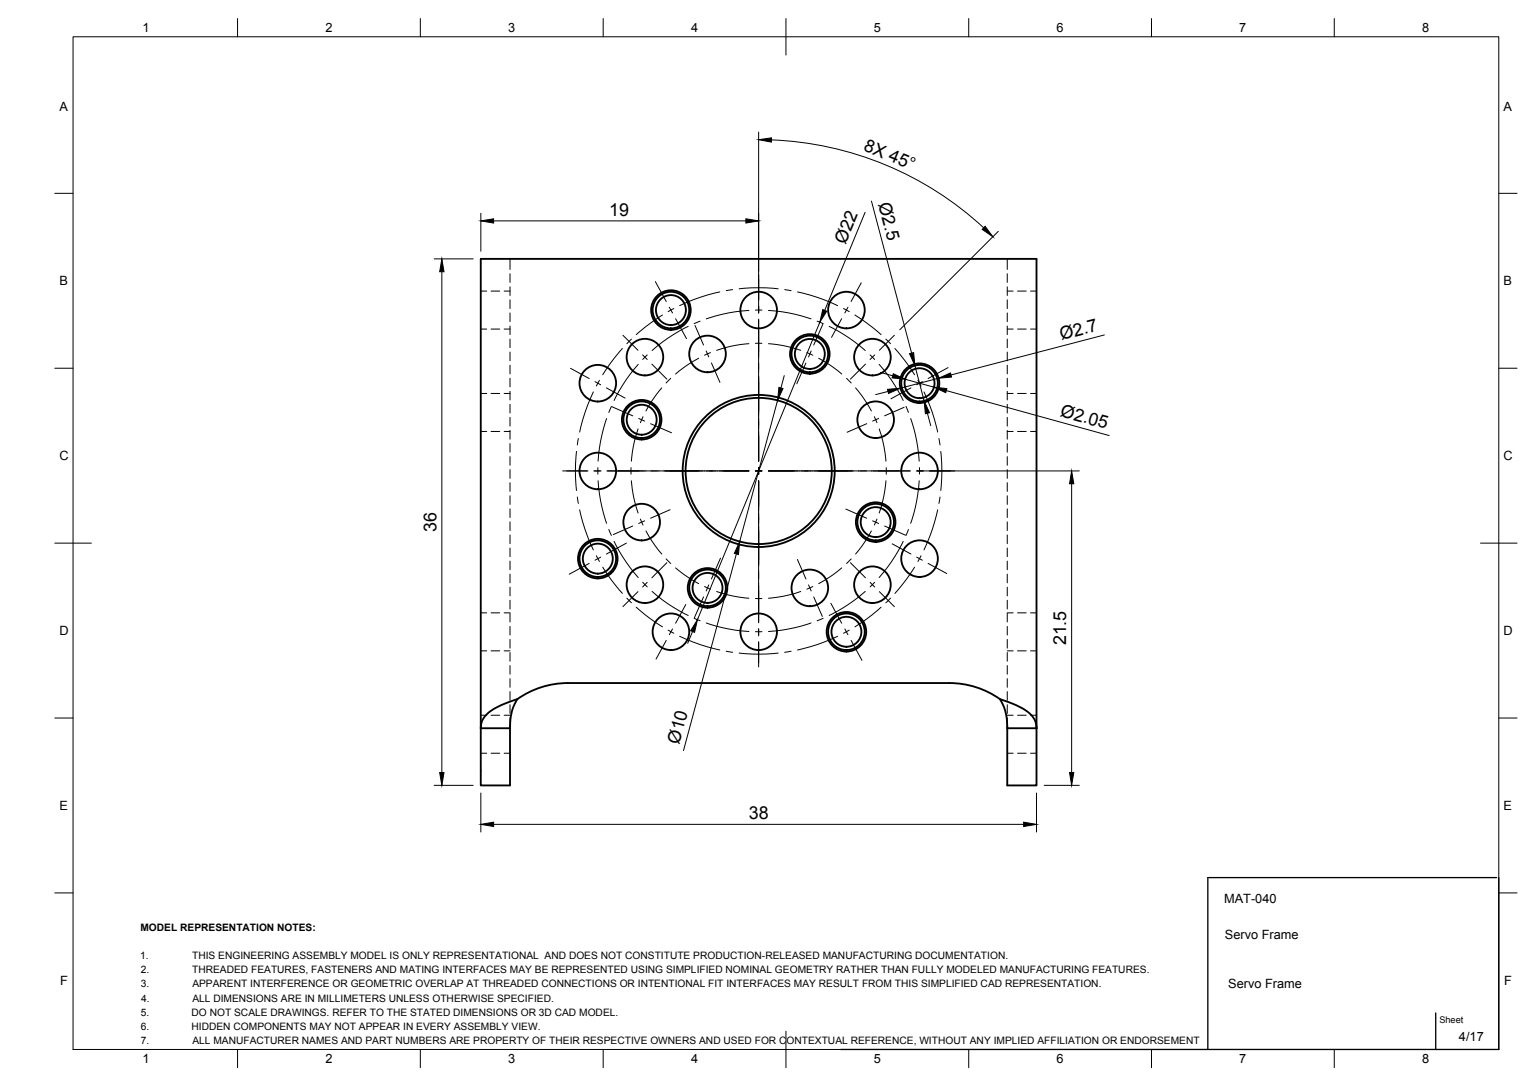
ISO-10303-21;
HEADER;
/* Generated by software containing ST-Developer
 * from STEP Tools, Inc. (www.steptools.com) 
 */

FILE_DESCRIPTION(
/* description */ ('STEP AP214'),
/* implementation_level */ '2;1');

FILE_NAME(
/* name */ 'Servo Frame.step',
/* time_stamp */ '2026-11-14T21:53:28-08:00',
/* author */ (''),
/* organization */ (''),
/* preprocessor_version */ 'ST-DEVELOPER v20.2',
/* originating_system */ 'Autodesk Translation Framework v15.17.0.0',
/* authorisation */ '');

FILE_SCHEMA (('AUTOMOTIVE_DESIGN { 1 0 10303 214 3 1 1 }'));
ENDSEC;

DATA;
#10=MECHANICAL_DESIGN_GEOMETRIC_PRESENTATION_REPRESENTATION('',(#320,#321,#322,#323,#324,#325,#326,#327,#328),#20176);
#187=OPEN_SHELL('',(#10781));
#188=OPEN_SHELL('',(#10782));
#189=OPEN_SHELL('',(#10783));
#190=OPEN_SHELL('',(#10784));
#191=OPEN_SHELL('',(#10785));
#192=OPEN_SHELL('',(#10786));
#193=OPEN_SHELL('',(#10787));
#194=OPEN_SHELL('',(#10788));
#195=SHELL_BASED_SURFACE_MODEL('Body2',(#187));
#196=SHELL_BASED_SURFACE_MODEL('Body3',(#188));
#197=SHELL_BASED_SURFACE_MODEL('Body4',(#189));
#198=SHELL_BASED_SURFACE_MODEL('Body5',(#190));
#199=SHELL_BASED_SURFACE_MODEL('Body6',(#191));
#200=SHELL_BASED_SURFACE_MODEL('Body7',(#192));
#201=SHELL_BASED_SURFACE_MODEL('Body8',(#193));
#202=SHELL_BASED_SURFACE_MODEL('Body9',(#194));
#203=ELLIPSE('',#11797,7.14648376237048,6.18893462761436);
#204=ELLIPSE('',#11803,7.14646345436459,6.18889945302544);
#205=CONICAL_SURFACE('',#11750,1.34999999991669,0.785398163397448);
#206=CONICAL_SURFACE('',#11752,1.34999999991669,0.785398163397448);
#207=CONICAL_SURFACE('',#11754,1.34999999991669,0.785398163397448);
#208=CONICAL_SURFACE('',#11756,1.34999999991669,0.785398163397448);
#209=CONICAL_SURFACE('',#11758,1.34999999990714,0.785398163397448);
#210=CONICAL_SURFACE('',#11760,1.34999999990714,0.785398163397448);
#211=CONICAL_SURFACE('',#11762,1.34999999990714,0.785398163397448);
#212=CONICAL_SURFACE('',#11764,1.34999999990714,0.785398163397448);
#213=CONICAL_SURFACE('',#11766,5.19997115839037,0.785393345879516);
#240=B_SPLINE_SURFACE_WITH_KNOTS('',3,3,((#19092,#19093,#19094,#19095),
(#19096,#19097,#19098,#19099),(#19100,#19101,#19102,#19103),(#19104,#19105,
#19106,#19107),(#19108,#19109,#19110,#19111),(#19112,#19113,#19114,#19115),
(#19116,#19117,#19118,#19119),(#19120,#19121,#19122,#19123),(#19124,#19125,
#19126,#19127)),.UNSPECIFIED.,.F.,.F.,.F.,(4,1,1,1,1,1,4),(4,4),(-0.01838458257717,
0.,0.25,0.5,0.75,1.,1.018710256812),(-0.03706965294501,1.037304298792),
 .UNSPECIFIED.);
#241=B_SPLINE_SURFACE_WITH_KNOTS('',3,3,((#19144,#19145,#19146,#19147),
(#19148,#19149,#19150,#19151),(#19152,#19153,#19154,#19155),(#19156,#19157,
#19158,#19159),(#19160,#19161,#19162,#19163),(#19164,#19165,#19166,#19167),
(#19168,#19169,#19170,#19171),(#19172,#19173,#19174,#19175),(#19176,#19177,
#19178,#19179)),.UNSPECIFIED.,.F.,.F.,.F.,(4,1,1,1,1,1,4),(4,4),(-0.01864501026175,
0.,0.25,0.5,0.75,1.,1.018470834436),(-0.03706965294501,1.037304298792),
 .UNSPECIFIED.);
#242=B_SPLINE_SURFACE_WITH_KNOTS('',3,3,((#19239,#19240,#19241,#19242),
(#19243,#19244,#19245,#19246),(#19247,#19248,#19249,#19250),(#19251,#19252,
#19253,#19254),(#19255,#19256,#19257,#19258),(#19259,#19260,#19261,#19262)),
 .UNSPECIFIED.,.F.,.F.,.F.,(4,1,1,4),(4,4),(-0.7776806408489,0.,1.,1.777680640849),
(-0.03706965294501,1.037069667454),.UNSPECIFIED.);
#243=B_SPLINE_SURFACE_WITH_KNOTS('',3,3,((#19263,#19264,#19265,#19266),
(#19267,#19268,#19269,#19270),(#19271,#19272,#19273,#19274),(#19275,#19276,
#19277,#19278),(#19279,#19280,#19281,#19282),(#19283,#19284,#19285,#19286)),
 .UNSPECIFIED.,.F.,.F.,.F.,(4,1,1,4),(4,4),(-0.7776806408488,0.,1.,1.777680640849),
(-0.03706965294501,1.037069667454),.UNSPECIFIED.);
#288=B_SPLINE_CURVE_WITH_KNOTS('',3,(#19003,#19004,#19005,#19006,#19007,
#19008,#19009,#19010,#19011,#19012,#19013,#19014,#19015,#19016),
 .UNSPECIFIED.,.F.,.F.,(4,2,2,2,2,2,4),(1.0000000090833E-6,0.0397704331538061,
0.0783295476556165,0.10311510516028,0.130769699028325,0.170261252779255,
0.207364811990595),.UNSPECIFIED.);
#289=B_SPLINE_CURVE_WITH_KNOTS('',3,(#19045,#19046,#19047,#19048,#19049,
#19050,#19051,#19052,#19053,#19054,#19055,#19056,#19057,#19058),
 .UNSPECIFIED.,.F.,.F.,(4,2,2,2,2,2,4),(1.00000005137352E-6,0.0364150080452644,
0.0751701681205766,0.102306577132939,0.126714048144896,0.164687443503408,
0.20385265381537),.UNSPECIFIED.);
#290=B_SPLINE_CURVE_WITH_KNOTS('',3,(#19129,#19130,#19131,#19132,#19133,
#19134,#19135,#19136,#19137,#19138,#19139,#19140,#19141,#19142),
 .UNSPECIFIED.,.F.,.F.,(4,2,2,2,2,2,4),(1.00000002985316E-6,0.0497274416726429,
0.101777541549185,0.213706159601663,0.317575823833734,0.371841554247195,
0.427578702498277),.UNSPECIFIED.);
#291=B_SPLINE_CURVE_WITH_KNOTS('',3,(#19182,#19183,#19184,#19185,#19186,
#19187,#19188,#19189,#19190,#19191,#19192,#19193,#19194,#19195),
 .UNSPECIFIED.,.F.,.F.,(4,2,2,2,2,2,4),(1.00000005253209E-6,0.0558510119021626,
0.110229405327848,0.214323647321834,0.326650579970185,0.379079827251892,
0.429160855957136),.UNSPECIFIED.);
#296=SHAPE_REPRESENTATION_RELATIONSHIP('SRR','None',#20258,#308);
#308=ADVANCED_BREP_SHAPE_REPRESENTATION('',(#355),#20164);
#320=STYLED_ITEM('',(#20334),#355);
#321=STYLED_ITEM('',(#20334),#195);
#322=STYLED_ITEM('',(#20334),#196);
#323=STYLED_ITEM('',(#20334),#197);
#324=STYLED_ITEM('',(#20334),#198);
#325=STYLED_ITEM('',(#20334),#199);
#326=STYLED_ITEM('',(#20334),#200);
#327=STYLED_ITEM('',(#20334),#201);
#328=STYLED_ITEM('',(#20334),#202);
#355=MANIFOLD_SOLID_BREP('Body1',#10946);
#450=FACE_BOUND('',#1962,.T.);
#451=FACE_BOUND('',#1963,.T.);
#452=FACE_BOUND('',#1964,.T.);
#453=FACE_BOUND('',#1965,.T.);
#454=FACE_BOUND('',#1966,.T.);
#455=FACE_BOUND('',#1967,.T.);
#456=FACE_BOUND('',#1968,.T.);
#457=FACE_BOUND('',#1969,.T.);
#458=FACE_BOUND('',#1970,.T.);
#459=FACE_BOUND('',#1971,.T.);
#460=FACE_BOUND('',#1972,.T.);
#461=FACE_BOUND('',#1973,.T.);
#462=FACE_BOUND('',#1974,.T.);
#463=FACE_BOUND('',#1975,.T.);
#464=FACE_BOUND('',#1976,.T.);
#465=FACE_BOUND('',#1977,.T.);
#466=FACE_BOUND('',#1978,.T.);
#467=FACE_BOUND('',#1979,.T.);
#468=FACE_BOUND('',#1980,.T.);
#469=FACE_BOUND('',#1981,.T.);
#470=FACE_BOUND('',#1982,.T.);
#471=FACE_BOUND('',#1983,.T.);
#472=FACE_BOUND('',#1984,.T.);
#473=FACE_BOUND('',#1985,.T.);
#474=FACE_BOUND('',#1986,.T.);
#475=FACE_BOUND('',#1994,.T.);
#476=FACE_BOUND('',#1995,.T.);
#477=FACE_BOUND('',#1996,.T.);
#478=FACE_BOUND('',#1997,.T.);
#479=FACE_BOUND('',#1998,.T.);
#480=FACE_BOUND('',#1999,.T.);
#481=FACE_BOUND('',#2000,.T.);
#482=FACE_BOUND('',#2001,.T.);
#483=FACE_BOUND('',#2002,.T.);
#484=FACE_BOUND('',#2003,.T.);
#485=FACE_BOUND('',#2004,.T.);
#486=FACE_BOUND('',#2005,.T.);
#487=FACE_BOUND('',#2006,.T.);
#488=FACE_BOUND('',#2007,.T.);
#489=FACE_BOUND('',#2008,.T.);
#490=FACE_BOUND('',#2009,.T.);
#491=FACE_BOUND('',#2010,.T.);
#492=FACE_BOUND('',#2011,.T.);
#493=FACE_BOUND('',#2012,.T.);
#494=FACE_BOUND('',#2013,.T.);
#495=FACE_BOUND('',#2014,.T.);
#496=FACE_BOUND('',#2015,.T.);
#497=FACE_BOUND('',#2016,.T.);
#498=FACE_BOUND('',#2017,.T.);
#499=FACE_BOUND('',#2018,.T.);
#500=FACE_BOUND('',#2020,.T.);
#501=FACE_BOUND('',#2021,.T.);
#502=FACE_BOUND('',#2022,.T.);
#503=FACE_BOUND('',#2023,.T.);
#504=FACE_BOUND('',#2027,.T.);
#505=FACE_BOUND('',#2028,.T.);
#506=FACE_BOUND('',#2029,.T.);
#507=FACE_BOUND('',#2030,.T.);
#508=FACE_BOUND('',#2046,.T.);
#509=FACE_BOUND('',#2047,.T.);
#510=FACE_BOUND('',#2048,.T.);
#511=FACE_BOUND('',#2049,.T.);
#512=FACE_BOUND('',#2051,.T.);
#513=FACE_BOUND('',#2052,.T.);
#514=FACE_BOUND('',#2053,.T.);
#515=FACE_BOUND('',#2054,.T.);
#808=PLANE('',#11792);
#809=PLANE('',#11798);
#810=PLANE('',#11806);
#811=PLANE('',#11809);
#812=PLANE('',#11810);
#813=PLANE('',#11814);
#814=PLANE('',#11822);
#815=PLANE('',#11827);
#816=PLANE('',#11830);
#817=PLANE('',#11835);
#818=PLANE('',#11838);
#819=PLANE('',#11839);
#820=PLANE('',#11840);
#821=PLANE('',#11841);
#1257=FACE_OUTER_BOUND('',#1919,.T.);
#1258=FACE_OUTER_BOUND('',#1920,.T.);
#1259=FACE_OUTER_BOUND('',#1921,.T.);
#1260=FACE_OUTER_BOUND('',#1922,.T.);
#1261=FACE_OUTER_BOUND('',#1923,.T.);
#1262=FACE_OUTER_BOUND('',#1924,.T.);
#1263=FACE_OUTER_BOUND('',#1925,.T.);
#1264=FACE_OUTER_BOUND('',#1926,.T.);
#1265=FACE_OUTER_BOUND('',#1927,.T.);
#1266=FACE_OUTER_BOUND('',#1928,.T.);
#1267=FACE_OUTER_BOUND('',#1929,.T.);
#1268=FACE_OUTER_BOUND('',#1930,.T.);
#1269=FACE_OUTER_BOUND('',#1931,.T.);
#1270=FACE_OUTER_BOUND('',#1932,.T.);
#1271=FACE_OUTER_BOUND('',#1933,.T.);
#1272=FACE_OUTER_BOUND('',#1934,.T.);
#1273=FACE_OUTER_BOUND('',#1935,.T.);
#1274=FACE_OUTER_BOUND('',#1936,.T.);
#1275=FACE_OUTER_BOUND('',#1937,.T.);
#1276=FACE_OUTER_BOUND('',#1938,.T.);
#1277=FACE_OUTER_BOUND('',#1939,.T.);
#1278=FACE_OUTER_BOUND('',#1940,.T.);
#1279=FACE_OUTER_BOUND('',#1941,.T.);
#1280=FACE_OUTER_BOUND('',#1942,.T.);
#1281=FACE_OUTER_BOUND('',#1943,.T.);
#1282=FACE_OUTER_BOUND('',#1944,.T.);
#1283=FACE_OUTER_BOUND('',#1945,.T.);
#1284=FACE_OUTER_BOUND('',#1946,.T.);
#1285=FACE_OUTER_BOUND('',#1947,.T.);
#1286=FACE_OUTER_BOUND('',#1948,.T.);
#1287=FACE_OUTER_BOUND('',#1949,.T.);
#1288=FACE_OUTER_BOUND('',#1950,.T.);
#1289=FACE_OUTER_BOUND('',#1951,.T.);
#1290=FACE_OUTER_BOUND('',#1952,.T.);
#1291=FACE_OUTER_BOUND('',#1953,.T.);
#1292=FACE_OUTER_BOUND('',#1954,.T.);
#1293=FACE_OUTER_BOUND('',#1955,.T.);
#1294=FACE_OUTER_BOUND('',#1956,.T.);
#1295=FACE_OUTER_BOUND('',#1957,.T.);
#1296=FACE_OUTER_BOUND('',#1958,.T.);
#1297=FACE_OUTER_BOUND('',#1959,.T.);
#1298=FACE_OUTER_BOUND('',#1960,.T.);
#1299=FACE_OUTER_BOUND('',#1961,.T.);
#1300=FACE_OUTER_BOUND('',#1987,.T.);
#1301=FACE_OUTER_BOUND('',#1988,.T.);
#1302=FACE_OUTER_BOUND('',#1989,.T.);
#1303=FACE_OUTER_BOUND('',#1990,.T.);
#1304=FACE_OUTER_BOUND('',#1991,.T.);
#1305=FACE_OUTER_BOUND('',#1992,.T.);
#1306=FACE_OUTER_BOUND('',#1993,.T.);
#1307=FACE_OUTER_BOUND('',#2019,.T.);
#1308=FACE_OUTER_BOUND('',#2024,.T.);
#1309=FACE_OUTER_BOUND('',#2025,.T.);
#1310=FACE_OUTER_BOUND('',#2026,.T.);
#1311=FACE_OUTER_BOUND('',#2031,.T.);
#1312=FACE_OUTER_BOUND('',#2032,.T.);
#1313=FACE_OUTER_BOUND('',#2033,.T.);
#1314=FACE_OUTER_BOUND('',#2034,.T.);
#1315=FACE_OUTER_BOUND('',#2035,.T.);
#1316=FACE_OUTER_BOUND('',#2036,.T.);
#1317=FACE_OUTER_BOUND('',#2037,.T.);
#1318=FACE_OUTER_BOUND('',#2038,.T.);
#1319=FACE_OUTER_BOUND('',#2039,.T.);
#1320=FACE_OUTER_BOUND('',#2040,.T.);
#1321=FACE_OUTER_BOUND('',#2041,.T.);
#1322=FACE_OUTER_BOUND('',#2042,.T.);
#1323=FACE_OUTER_BOUND('',#2043,.T.);
#1324=FACE_OUTER_BOUND('',#2044,.T.);
#1325=FACE_OUTER_BOUND('',#2045,.T.);
#1326=FACE_OUTER_BOUND('',#2050,.T.);
#1327=FACE_OUTER_BOUND('',#2055,.T.);
#1328=FACE_OUTER_BOUND('',#2056,.T.);
#1329=FACE_OUTER_BOUND('',#2057,.T.);
#1330=FACE_OUTER_BOUND('',#2058,.T.);
#1331=FACE_OUTER_BOUND('',#2059,.T.);
#1332=FACE_OUTER_BOUND('',#2060,.T.);
#1333=FACE_OUTER_BOUND('',#2061,.T.);
#1334=FACE_OUTER_BOUND('',#2062,.T.);
#1335=FACE_OUTER_BOUND('',#2063,.T.);
#1336=FACE_OUTER_BOUND('',#2064,.T.);
#1919=EDGE_LOOP('',(#9045,#9046,#9047,#9048));
#1920=EDGE_LOOP('',(#9049,#9050,#9051,#9052));
#1921=EDGE_LOOP('',(#9053,#9054,#9055,#9056));
#1922=EDGE_LOOP('',(#9057,#9058,#9059,#9060));
#1923=EDGE_LOOP('',(#9061,#9062,#9063,#9064));
#1924=EDGE_LOOP('',(#9065,#9066,#9067,#9068));
#1925=EDGE_LOOP('',(#9069,#9070,#9071,#9072));
#1926=EDGE_LOOP('',(#9073,#9074,#9075,#9076));
#1927=EDGE_LOOP('',(#9077,#9078,#9079,#9080));
#1928=EDGE_LOOP('',(#9081,#9082,#9083,#9084));
#1929=EDGE_LOOP('',(#9085,#9086,#9087,#9088));
#1930=EDGE_LOOP('',(#9089,#9090,#9091,#9092));
#1931=EDGE_LOOP('',(#9093,#9094,#9095,#9096));
#1932=EDGE_LOOP('',(#9097,#9098,#9099,#9100));
#1933=EDGE_LOOP('',(#9101,#9102,#9103,#9104));
#1934=EDGE_LOOP('',(#9105,#9106,#9107,#9108));
#1935=EDGE_LOOP('',(#9109,#9110,#9111,#9112));
#1936=EDGE_LOOP('',(#9113,#9114,#9115,#9116));
#1937=EDGE_LOOP('',(#9117,#9118,#9119,#9120));
#1938=EDGE_LOOP('',(#9121,#9122,#9123,#9124));
#1939=EDGE_LOOP('',(#9125,#9126,#9127,#9128));
#1940=EDGE_LOOP('',(#9129,#9130,#9131,#9132));
#1941=EDGE_LOOP('',(#9133,#9134,#9135,#9136));
#1942=EDGE_LOOP('',(#9137,#9138,#9139,#9140));
#1943=EDGE_LOOP('',(#9141,#9142,#9143,#9144));
#1944=EDGE_LOOP('',(#9145,#9146,#9147,#9148));
#1945=EDGE_LOOP('',(#9149,#9150,#9151,#9152));
#1946=EDGE_LOOP('',(#9153,#9154,#9155,#9156));
#1947=EDGE_LOOP('',(#9157,#9158,#9159,#9160));
#1948=EDGE_LOOP('',(#9161,#9162,#9163,#9164));
#1949=EDGE_LOOP('',(#9165,#9166,#9167,#9168));
#1950=EDGE_LOOP('',(#9169,#9170,#9171,#9172));
#1951=EDGE_LOOP('',(#9173,#9174,#9175,#9176));
#1952=EDGE_LOOP('',(#9177,#9178,#9179,#9180));
#1953=EDGE_LOOP('',(#9181,#9182,#9183,#9184));
#1954=EDGE_LOOP('',(#9185,#9186,#9187,#9188));
#1955=EDGE_LOOP('',(#9189,#9190,#9191,#9192));
#1956=EDGE_LOOP('',(#9193,#9194,#9195,#9196));
#1957=EDGE_LOOP('',(#9197,#9198,#9199,#9200));
#1958=EDGE_LOOP('',(#9201,#9202,#9203,#9204));
#1959=EDGE_LOOP('',(#9205,#9206,#9207,#9208));
#1960=EDGE_LOOP('',(#9209,#9210,#9211,#9212));
#1961=EDGE_LOOP('',(#9213,#9214,#9215,#9216,#9217,#9218));
#1962=EDGE_LOOP('',(#9219));
#1963=EDGE_LOOP('',(#9220));
#1964=EDGE_LOOP('',(#9221));
#1965=EDGE_LOOP('',(#9222));
#1966=EDGE_LOOP('',(#9223));
#1967=EDGE_LOOP('',(#9224));
#1968=EDGE_LOOP('',(#9225));
#1969=EDGE_LOOP('',(#9226));
#1970=EDGE_LOOP('',(#9227));
#1971=EDGE_LOOP('',(#9228));
#1972=EDGE_LOOP('',(#9229));
#1973=EDGE_LOOP('',(#9230));
#1974=EDGE_LOOP('',(#9231));
#1975=EDGE_LOOP('',(#9232));
#1976=EDGE_LOOP('',(#9233));
#1977=EDGE_LOOP('',(#9234));
#1978=EDGE_LOOP('',(#9235));
#1979=EDGE_LOOP('',(#9236));
#1980=EDGE_LOOP('',(#9237));
#1981=EDGE_LOOP('',(#9238));
#1982=EDGE_LOOP('',(#9239));
#1983=EDGE_LOOP('',(#9240));
#1984=EDGE_LOOP('',(#9241));
#1985=EDGE_LOOP('',(#9242));
#1986=EDGE_LOOP('',(#9243));
#1987=EDGE_LOOP('',(#9244,#9245,#9246,#9247,#9248));
#1988=EDGE_LOOP('',(#9249,#9250,#9251,#9252,#9253,#9254,#9255,#9256,#9257,
#9258,#9259,#9260));
#1989=EDGE_LOOP('',(#9261,#9262,#9263,#9264,#9265));
#1990=EDGE_LOOP('',(#9266,#9267,#9268,#9269,#9270));
#1991=EDGE_LOOP('',(#9271,#9272,#9273,#9274));
#1992=EDGE_LOOP('',(#9275,#9276,#9277,#9278,#9279));
#1993=EDGE_LOOP('',(#9280,#9281,#9282,#9283,#9284,#9285));
#1994=EDGE_LOOP('',(#9286));
#1995=EDGE_LOOP('',(#9287));
#1996=EDGE_LOOP('',(#9288));
#1997=EDGE_LOOP('',(#9289));
#1998=EDGE_LOOP('',(#9290));
#1999=EDGE_LOOP('',(#9291));
#2000=EDGE_LOOP('',(#9292));
#2001=EDGE_LOOP('',(#9293));
#2002=EDGE_LOOP('',(#9294));
#2003=EDGE_LOOP('',(#9295));
#2004=EDGE_LOOP('',(#9296));
#2005=EDGE_LOOP('',(#9297));
#2006=EDGE_LOOP('',(#9298));
#2007=EDGE_LOOP('',(#9299));
#2008=EDGE_LOOP('',(#9300));
#2009=EDGE_LOOP('',(#9301));
#2010=EDGE_LOOP('',(#9302));
#2011=EDGE_LOOP('',(#9303));
#2012=EDGE_LOOP('',(#9304));
#2013=EDGE_LOOP('',(#9305));
#2014=EDGE_LOOP('',(#9306));
#2015=EDGE_LOOP('',(#9307));
#2016=EDGE_LOOP('',(#9308));
#2017=EDGE_LOOP('',(#9309));
#2018=EDGE_LOOP('',(#9310));
#2019=EDGE_LOOP('',(#9311,#9312,#9313,#9314,#9315,#9316,#9317,#9318));
#2020=EDGE_LOOP('',(#9319));
#2021=EDGE_LOOP('',(#9320));
#2022=EDGE_LOOP('',(#9321));
#2023=EDGE_LOOP('',(#9322));
#2024=EDGE_LOOP('',(#9323,#9324,#9325,#9326,#9327));
#2025=EDGE_LOOP('',(#9328,#9329,#9330,#9331,#9332));
#2026=EDGE_LOOP('',(#9333,#9334,#9335,#9336,#9337,#9338,#9339,#9340));
#2027=EDGE_LOOP('',(#9341));
#2028=EDGE_LOOP('',(#9342));
#2029=EDGE_LOOP('',(#9343));
#2030=EDGE_LOOP('',(#9344));
#2031=EDGE_LOOP('',(#9345,#9346,#9347,#9348,#9349));
#2032=EDGE_LOOP('',(#9350,#9351,#9352,#9353,#9354));
#2033=EDGE_LOOP('',(#9355,#9356,#9357,#9358,#9359));
#2034=EDGE_LOOP('',(#9360,#9361,#9362,#9363));
#2035=EDGE_LOOP('',(#9364,#9365,#9366,#9367));
#2036=EDGE_LOOP('',(#9368,#9369,#9370,#9371));
#2037=EDGE_LOOP('',(#9372,#9373,#9374,#9375));
#2038=EDGE_LOOP('',(#9376,#9377,#9378,#9379,#9380));
#2039=EDGE_LOOP('',(#9381,#9382,#9383,#9384,#9385));
#2040=EDGE_LOOP('',(#9386,#9387,#9388,#9389));
#2041=EDGE_LOOP('',(#9390,#9391,#9392,#9393));
#2042=EDGE_LOOP('',(#9394,#9395,#9396,#9397));
#2043=EDGE_LOOP('',(#9398,#9399,#9400,#9401,#9402));
#2044=EDGE_LOOP('',(#9403,#9404,#9405,#9406));
#2045=EDGE_LOOP('',(#9407,#9408,#9409,#9410,#9411,#9412,#9413,#9414));
#2046=EDGE_LOOP('',(#9415));
#2047=EDGE_LOOP('',(#9416));
#2048=EDGE_LOOP('',(#9417));
#2049=EDGE_LOOP('',(#9418));
#2050=EDGE_LOOP('',(#9419,#9420,#9421,#9422,#9423,#9424,#9425,#9426));
#2051=EDGE_LOOP('',(#9427));
#2052=EDGE_LOOP('',(#9428));
#2053=EDGE_LOOP('',(#9429));
#2054=EDGE_LOOP('',(#9430));
#2055=EDGE_LOOP('',(#9431,#9432,#9433,#9434));
#2056=EDGE_LOOP('',(#9435,#9436,#9437,#9438));
#2057=EDGE_LOOP('',(#9439,#9440,#9441,#9442));
#2058=EDGE_LOOP('',(#9443,#9444,#9445,#9446));
#2059=EDGE_LOOP('',(#9447,#9448,#9449,#9450));
#2060=EDGE_LOOP('',(#9451,#9452,#9453,#9454));
#2061=EDGE_LOOP('',(#9455,#9456,#9457,#9458));
#2062=EDGE_LOOP('',(#9459,#9460,#9461,#9462));
#2063=EDGE_LOOP('',(#9463,#9464,#9465,#9466));
#2064=EDGE_LOOP('',(#9467,#9468,#9469,#9470));
#2967=LINE('',#18756,#3955);
#2968=LINE('',#18762,#3956);
#2969=LINE('',#18768,#3957);
#2970=LINE('',#18774,#3958);
#2971=LINE('',#18780,#3959);
#2972=LINE('',#18786,#3960);
#2973=LINE('',#18792,#3961);
#2974=LINE('',#18798,#3962);
#2975=LINE('',#18804,#3963);
#2976=LINE('',#18810,#3964);
#2977=LINE('',#18816,#3965);
#2978=LINE('',#18822,#3966);
#2979=LINE('',#18828,#3967);
#2980=LINE('',#18834,#3968);
#2981=LINE('',#18840,#3969);
#2982=LINE('',#18846,#3970);
#2983=LINE('',#18852,#3971);
#2984=LINE('',#18858,#3972);
#2985=LINE('',#18864,#3973);
#2986=LINE('',#18870,#3974);
#2987=LINE('',#18876,#3975);
#2988=LINE('',#18882,#3976);
#2989=LINE('',#18888,#3977);
#2990=LINE('',#18894,#3978);
#2991=LINE('',#18900,#3979);
#2992=LINE('',#18904,#3980);
#2993=LINE('',#18908,#3981);
#2994=LINE('',#18912,#3982);
#2995=LINE('',#18916,#3983);
#2996=LINE('',#18920,#3984);
#2997=LINE('',#18924,#3985);
#2998=LINE('',#18928,#3986);
#2999=LINE('',#18932,#3987);
#3000=LINE('',#18936,#3988);
#3001=LINE('',#18942,#3989);
#3002=LINE('',#18948,#3990);
#3003=LINE('',#18954,#3991);
#3004=LINE('',#18960,#3992);
#3005=LINE('',#18966,#3993);
#3006=LINE('',#18972,#3994);
#3007=LINE('',#18978,#3995);
#3008=LINE('',#18984,#3996);
#3009=LINE('',#18989,#3997);
#3010=LINE('',#18991,#3998);
#3011=LINE('',#18995,#3999);
#3012=LINE('',#18998,#4000);
#3013=LINE('',#19019,#4001);
#3014=LINE('',#19022,#4002);
#3015=LINE('',#19024,#4003);
#3016=LINE('',#19026,#4004);
#3017=LINE('',#19030,#4005);
#3018=LINE('',#19034,#4006);
#3019=LINE('',#19036,#4007);
#3020=LINE('',#19038,#4008);
#3021=LINE('',#19042,#4009);
#3022=LINE('',#19061,#4010);
#3023=LINE('',#19063,#4011);
#3024=LINE('',#19066,#4012);
#3025=LINE('',#19069,#4013);
#3026=LINE('',#19070,#4014);
#3027=LINE('',#19075,#4015);
#3028=LINE('',#19076,#4016);
#3029=LINE('',#19078,#4017);
#3030=LINE('',#19079,#4018);
#3031=LINE('',#19082,#4019);
#3032=LINE('',#19086,#4020);
#3033=LINE('',#19090,#4021);
#3034=LINE('',#19143,#4022);
#3035=LINE('',#19181,#4023);
#3036=LINE('',#19201,#4024);
#3037=LINE('',#19204,#4025);
#3038=LINE('',#19207,#4026);
#3039=LINE('',#19210,#4027);
#3040=LINE('',#19215,#4028);
#3041=LINE('',#19218,#4029);
#3042=LINE('',#19219,#4030);
#3043=LINE('',#19221,#4031);
#3044=LINE('',#19222,#4032);
#3045=LINE('',#19226,#4033);
#3046=LINE('',#19229,#4034);
#3047=LINE('',#19232,#4035);
#3048=LINE('',#19235,#4036);
#3049=LINE('',#19236,#4037);
#3050=LINE('',#19288,#4038);
#3051=LINE('',#19289,#4039);
#3052=LINE('',#19292,#4040);
#3053=LINE('',#19294,#4041);
#3054=LINE('',#19295,#4042);
#3055=LINE('',#19299,#4043);
#3056=LINE('',#19302,#4044);
#3057=LINE('',#19305,#4045);
#3058=LINE('',#19307,#4046);
#3059=LINE('',#19311,#4047);
#3060=LINE('',#19313,#4048);
#3061=LINE('',#19320,#4049);
#3062=LINE('',#19326,#4050);
#3063=LINE('',#19332,#4051);
#3064=LINE('',#19338,#4052);
#3065=LINE('',#19344,#4053);
#3066=LINE('',#19350,#4054);
#3067=LINE('',#19356,#4055);
#3068=LINE('',#19362,#4056);
#3955=VECTOR('',#14047,1.25);
#3956=VECTOR('',#14054,1.25);
#3957=VECTOR('',#14061,1.25);
#3958=VECTOR('',#14068,1.25);
#3959=VECTOR('',#14075,1.025);
#3960=VECTOR('',#14082,1.025);
#3961=VECTOR('',#14089,1.025);
#3962=VECTOR('',#14096,1.025);
#3963=VECTOR('',#14103,1.25);
#3964=VECTOR('',#14110,1.25);
#3965=VECTOR('',#14117,1.25);
#3966=VECTOR('',#14124,1.25);
#3967=VECTOR('',#14131,1.025);
#3968=VECTOR('',#14138,1.025);
#3969=VECTOR('',#14145,1.025);
#3970=VECTOR('',#14152,1.025);
#3971=VECTOR('',#14159,1.25);
#3972=VECTOR('',#14166,1.25);
#3973=VECTOR('',#14173,1.25);
#3974=VECTOR('',#14180,1.25);
#3975=VECTOR('',#14187,1.25);
#3976=VECTOR('',#14194,1.25);
#3977=VECTOR('',#14201,1.25);
#3978=VECTOR('',#14208,1.25);
#3979=VECTOR('',#14215,5.);
#3980=VECTOR('',#14220,1.34999999991669);
#3981=VECTOR('',#14225,1.34999999991669);
#3982=VECTOR('',#14230,1.34999999991669);
#3983=VECTOR('',#14235,1.34999999991669);
#3984=VECTOR('',#14240,1.34999999990714);
#3985=VECTOR('',#14245,1.34999999990714);
#3986=VECTOR('',#14250,1.34999999990714);
#3987=VECTOR('',#14255,1.34999999990714);
#3988=VECTOR('',#14260,5.19997115839037);
#3989=VECTOR('',#14267,1.3);
#3990=VECTOR('',#14274,1.3);
#3991=VECTOR('',#14281,1.3);
#3992=VECTOR('',#14288,1.3);
#3993=VECTOR('',#14295,1.3);
#3994=VECTOR('',#14302,1.3);
#3995=VECTOR('',#14309,1.3);
#3996=VECTOR('',#14316,1.3);
#3997=VECTOR('',#14321,1000.);
#3998=VECTOR('',#14322,1000.);
#3999=VECTOR('',#14325,1000.);
#4000=VECTOR('',#14328,1000.);
#4001=VECTOR('',#14335,1000.);
#4002=VECTOR('',#14338,1000.);
#4003=VECTOR('',#14339,1000.);
#4004=VECTOR('',#14340,1000.);
#4005=VECTOR('',#14343,1000.);
#4006=VECTOR('',#14346,1000.);
#4007=VECTOR('',#14347,1000.);
#4008=VECTOR('',#14348,1000.);
#4009=VECTOR('',#14353,1000.);
#4010=VECTOR('',#14358,1000.);
#4011=VECTOR('',#14359,1000.);
#4012=VECTOR('',#14362,1000.);
#4013=VECTOR('',#14365,1000.);
#4014=VECTOR('',#14366,1000.);
#4015=VECTOR('',#14371,1000.);
#4016=VECTOR('',#14372,1000.);
#4017=VECTOR('',#14375,1000.);
#4018=VECTOR('',#14376,1000.);
#4019=VECTOR('',#14379,1000.);
#4020=VECTOR('',#14382,1000.);
#4021=VECTOR('',#14385,1000.);
#4022=VECTOR('',#14388,1000.);
#4023=VECTOR('',#14389,1000.);
#4024=VECTOR('',#14394,1000.);
#4025=VECTOR('',#14397,1000.);
#4026=VECTOR('',#14400,1000.);
#4027=VECTOR('',#14403,1000.);
#4028=VECTOR('',#14410,1000.);
#4029=VECTOR('',#14413,1000.);
#4030=VECTOR('',#14414,1000.);
#4031=VECTOR('',#14415,1000.);
#4032=VECTOR('',#14416,1000.);
#4033=VECTOR('',#14421,1000.);
#4034=VECTOR('',#14424,1000.);
#4035=VECTOR('',#14427,1000.);
#4036=VECTOR('',#14430,1000.);
#4037=VECTOR('',#14431,1000.);
#4038=VECTOR('',#14436,1000.);
#4039=VECTOR('',#14437,1000.);
#4040=VECTOR('',#14440,1000.);
#4041=VECTOR('',#14441,1000.);
#4042=VECTOR('',#14442,1000.);
#4043=VECTOR('',#14447,1000.);
#4044=VECTOR('',#14450,1000.);
#4045=VECTOR('',#14453,1000.);
#4046=VECTOR('',#14456,1000.);
#4047=VECTOR('',#14463,1000.);
#4048=VECTOR('',#14466,1000.);
#4049=VECTOR('',#14475,1.25);
#4050=VECTOR('',#14482,1.25);
#4051=VECTOR('',#14489,1.25);
#4052=VECTOR('',#14496,1.25);
#4053=VECTOR('',#14503,1.25);
#4054=VECTOR('',#14510,1.25);
#4055=VECTOR('',#14517,1.25);
#4056=VECTOR('',#14524,1.25);
#4476=CIRCLE('',#11676,1.25);
#4477=CIRCLE('',#11677,1.25);
#4478=CIRCLE('',#11679,1.25);
#4479=CIRCLE('',#11680,1.25);
#4480=CIRCLE('',#11682,1.25);
#4481=CIRCLE('',#11683,1.25);
#4482=CIRCLE('',#11685,1.25);
#4483=CIRCLE('',#11686,1.25);
#4484=CIRCLE('',#11688,1.025);
#4485=CIRCLE('',#11689,1.025);
#4486=CIRCLE('',#11691,1.025);
#4487=CIRCLE('',#11692,1.025);
#4488=CIRCLE('',#11694,1.025);
#4489=CIRCLE('',#11695,1.025);
#4490=CIRCLE('',#11697,1.025);
#4491=CIRCLE('',#11698,1.025);
#4492=CIRCLE('',#11700,1.25);
#4493=CIRCLE('',#11701,1.25);
#4494=CIRCLE('',#11703,1.25);
#4495=CIRCLE('',#11704,1.25);
#4496=CIRCLE('',#11706,1.25);
#4497=CIRCLE('',#11707,1.25);
#4498=CIRCLE('',#11709,1.25);
#4499=CIRCLE('',#11710,1.25);
#4500=CIRCLE('',#11712,1.025);
#4501=CIRCLE('',#11713,1.025);
#4502=CIRCLE('',#11715,1.025);
#4503=CIRCLE('',#11716,1.025);
#4504=CIRCLE('',#11718,1.025);
#4505=CIRCLE('',#11719,1.025);
#4506=CIRCLE('',#11721,1.025);
#4507=CIRCLE('',#11722,1.025);
#4508=CIRCLE('',#11724,1.25);
#4509=CIRCLE('',#11725,1.25);
#4510=CIRCLE('',#11727,1.25);
#4511=CIRCLE('',#11728,1.25);
#4512=CIRCLE('',#11730,1.25);
#4513=CIRCLE('',#11731,1.25);
#4514=CIRCLE('',#11733,1.25);
#4515=CIRCLE('',#11734,1.25);
#4516=CIRCLE('',#11736,1.25);
#4517=CIRCLE('',#11737,1.25);
#4518=CIRCLE('',#11739,1.25);
#4519=CIRCLE('',#11740,1.25);
#4520=CIRCLE('',#11742,1.25);
#4521=CIRCLE('',#11743,1.25);
#4522=CIRCLE('',#11745,1.25);
#4523=CIRCLE('',#11746,1.25);
#4524=CIRCLE('',#11748,5.);
#4525=CIRCLE('',#11749,5.);
#4526=CIRCLE('',#11751,1.35000000003038);
#4527=CIRCLE('',#11753,1.35000000003038);
#4528=CIRCLE('',#11755,1.35000000003038);
#4529=CIRCLE('',#11757,1.35000000003038);
#4530=CIRCLE('',#11759,1.35000000002083);
#4531=CIRCLE('',#11761,1.35000000002083);
#4532=CIRCLE('',#11763,1.35000000002083);
#4533=CIRCLE('',#11765,1.35000000002083);
#4534=CIRCLE('',#11767,5.19994989682595);
#4535=CIRCLE('',#11769,1.3);
#4536=CIRCLE('',#11770,1.3);
#4537=CIRCLE('',#11772,1.3);
#4538=CIRCLE('',#11773,1.3);
#4539=CIRCLE('',#11775,1.3);
#4540=CIRCLE('',#11776,1.3);
#4541=CIRCLE('',#11778,1.3);
#4542=CIRCLE('',#11779,1.3);
#4543=CIRCLE('',#11781,1.3);
#4544=CIRCLE('',#11782,1.3);
#4545=CIRCLE('',#11784,1.3);
#4546=CIRCLE('',#11785,1.3);
#4547=CIRCLE('',#11787,1.3);
#4548=CIRCLE('',#11788,1.3);
#4549=CIRCLE('',#11790,1.3);
#4550=CIRCLE('',#11791,1.3);
#4551=CIRCLE('',#11793,6.);
#4552=CIRCLE('',#11794,6.);
#4553=CIRCLE('',#11796,0.5);
#4554=CIRCLE('',#11799,2.5);
#4555=CIRCLE('',#11800,2.5);
#4556=CIRCLE('',#11801,0.5);
#4557=CIRCLE('',#11805,6.);
#4558=CIRCLE('',#11808,6.);
#4559=CIRCLE('',#11811,2.);
#4560=CIRCLE('',#11812,2.);
#4561=CIRCLE('',#11813,2.);
#4562=CIRCLE('',#11815,2.);
#4563=CIRCLE('',#11816,2.);
#4564=CIRCLE('',#11817,2.);
#4565=CIRCLE('',#11819,4.05035655858838);
#4566=CIRCLE('',#11821,4.0503565587057);
#4567=CIRCLE('',#11824,2.);
#4568=CIRCLE('',#11826,2.);
#4569=CIRCLE('',#11829,2.);
#4570=CIRCLE('',#11832,2.);
#4571=CIRCLE('',#11834,2.);
#4572=CIRCLE('',#11837,2.);
#4573=CIRCLE('',#11843,1.25);
#4574=CIRCLE('',#11844,1.25);
#4575=CIRCLE('',#11846,1.25);
#4576=CIRCLE('',#11847,1.25);
#4577=CIRCLE('',#11849,1.25);
#4578=CIRCLE('',#11850,1.25);
#4579=CIRCLE('',#11852,1.25);
#4580=CIRCLE('',#11853,1.25);
#4581=CIRCLE('',#11855,1.25);
#4582=CIRCLE('',#11856,1.25);
#4583=CIRCLE('',#11858,1.25);
#4584=CIRCLE('',#11859,1.25);
#4585=CIRCLE('',#11861,1.25);
#4586=CIRCLE('',#11862,1.25);
#4587=CIRCLE('',#11864,1.25);
#4588=CIRCLE('',#11865,1.25);
#5317=VERTEX_POINT('',#18753);
#5318=VERTEX_POINT('',#18755);
#5319=VERTEX_POINT('',#18759);
#5320=VERTEX_POINT('',#18761);
#5321=VERTEX_POINT('',#18765);
#5322=VERTEX_POINT('',#18767);
#5323=VERTEX_POINT('',#18771);
#5324=VERTEX_POINT('',#18773);
#5325=VERTEX_POINT('',#18777);
#5326=VERTEX_POINT('',#18779);
#5327=VERTEX_POINT('',#18783);
#5328=VERTEX_POINT('',#18785);
#5329=VERTEX_POINT('',#18789);
#5330=VERTEX_POINT('',#18791);
#5331=VERTEX_POINT('',#18795);
#5332=VERTEX_POINT('',#18797);
#5333=VERTEX_POINT('',#18801);
#5334=VERTEX_POINT('',#18803);
#5335=VERTEX_POINT('',#18807);
#5336=VERTEX_POINT('',#18809);
#5337=VERTEX_POINT('',#18813);
#5338=VERTEX_POINT('',#18815);
#5339=VERTEX_POINT('',#18819);
#5340=VERTEX_POINT('',#18821);
#5341=VERTEX_POINT('',#18825);
#5342=VERTEX_POINT('',#18827);
#5343=VERTEX_POINT('',#18831);
#5344=VERTEX_POINT('',#18833);
#5345=VERTEX_POINT('',#18837);
#5346=VERTEX_POINT('',#18839);
#5347=VERTEX_POINT('',#18843);
#5348=VERTEX_POINT('',#18845);
#5349=VERTEX_POINT('',#18849);
#5350=VERTEX_POINT('',#18851);
#5351=VERTEX_POINT('',#18855);
#5352=VERTEX_POINT('',#18857);
#5353=VERTEX_POINT('',#18861);
#5354=VERTEX_POINT('',#18863);
#5355=VERTEX_POINT('',#18867);
#5356=VERTEX_POINT('',#18869);
#5357=VERTEX_POINT('',#18873);
#5358=VERTEX_POINT('',#18875);
#5359=VERTEX_POINT('',#18879);
#5360=VERTEX_POINT('',#18881);
#5361=VERTEX_POINT('',#18885);
#5362=VERTEX_POINT('',#18887);
#5363=VERTEX_POINT('',#18891);
#5364=VERTEX_POINT('',#18893);
#5365=VERTEX_POINT('',#18897);
#5366=VERTEX_POINT('',#18899);
#5367=VERTEX_POINT('',#18903);
#5368=VERTEX_POINT('',#18907);
#5369=VERTEX_POINT('',#18911);
#5370=VERTEX_POINT('',#18915);
#5371=VERTEX_POINT('',#18919);
#5372=VERTEX_POINT('',#18923);
#5373=VERTEX_POINT('',#18927);
#5374=VERTEX_POINT('',#18931);
#5375=VERTEX_POINT('',#18935);
#5376=VERTEX_POINT('',#18939);
#5377=VERTEX_POINT('',#18941);
#5378=VERTEX_POINT('',#18945);
#5379=VERTEX_POINT('',#18947);
#5380=VERTEX_POINT('',#18951);
#5381=VERTEX_POINT('',#18953);
#5382=VERTEX_POINT('',#18957);
#5383=VERTEX_POINT('',#18959);
#5384=VERTEX_POINT('',#18963);
#5385=VERTEX_POINT('',#18965);
#5386=VERTEX_POINT('',#18969);
#5387=VERTEX_POINT('',#18971);
#5388=VERTEX_POINT('',#18975);
#5389=VERTEX_POINT('',#18977);
#5390=VERTEX_POINT('',#18981);
#5391=VERTEX_POINT('',#18983);
#5392=VERTEX_POINT('',#18987);
#5393=VERTEX_POINT('',#18988);
#5394=VERTEX_POINT('',#18990);
#5395=VERTEX_POINT('',#18992);
#5396=VERTEX_POINT('',#18994);
#5397=VERTEX_POINT('',#18996);
#5398=VERTEX_POINT('',#19000);
#5399=VERTEX_POINT('',#19002);
#5400=VERTEX_POINT('',#19017);
#5401=VERTEX_POINT('',#19021);
#5402=VERTEX_POINT('',#19023);
#5403=VERTEX_POINT('',#19025);
#5404=VERTEX_POINT('',#19027);
#5405=VERTEX_POINT('',#19029);
#5406=VERTEX_POINT('',#19031);
#5407=VERTEX_POINT('',#19033);
#5408=VERTEX_POINT('',#19035);
#5409=VERTEX_POINT('',#19037);
#5410=VERTEX_POINT('',#19041);
#5411=VERTEX_POINT('',#19043);
#5412=VERTEX_POINT('',#19060);
#5413=VERTEX_POINT('',#19062);
#5414=VERTEX_POINT('',#19064);
#5415=VERTEX_POINT('',#19068);
#5416=VERTEX_POINT('',#19072);
#5417=VERTEX_POINT('',#19074);
#5418=VERTEX_POINT('',#19081);
#5419=VERTEX_POINT('',#19083);
#5420=VERTEX_POINT('',#19085);
#5421=VERTEX_POINT('',#19087);
#5422=VERTEX_POINT('',#19089);
#5423=VERTEX_POINT('',#19128);
#5424=VERTEX_POINT('',#19180);
#5425=VERTEX_POINT('',#19197);
#5426=VERTEX_POINT('',#19198);
#5427=VERTEX_POINT('',#19200);
#5428=VERTEX_POINT('',#19202);
#5429=VERTEX_POINT('',#19205);
#5430=VERTEX_POINT('',#19209);
#5431=VERTEX_POINT('',#19213);
#5432=VERTEX_POINT('',#19217);
#5433=VERTEX_POINT('',#19220);
#5434=VERTEX_POINT('',#19224);
#5435=VERTEX_POINT('',#19228);
#5436=VERTEX_POINT('',#19230);
#5437=VERTEX_POINT('',#19234);
#5438=VERTEX_POINT('',#19287);
#5439=VERTEX_POINT('',#19291);
#5440=VERTEX_POINT('',#19293);
#5441=VERTEX_POINT('',#19297);
#5442=VERTEX_POINT('',#19301);
#5443=VERTEX_POINT('',#19303);
#5444=VERTEX_POINT('',#19317);
#5445=VERTEX_POINT('',#19319);
#5446=VERTEX_POINT('',#19323);
#5447=VERTEX_POINT('',#19325);
#5448=VERTEX_POINT('',#19329);
#5449=VERTEX_POINT('',#19331);
#5450=VERTEX_POINT('',#19335);
#5451=VERTEX_POINT('',#19337);
#5452=VERTEX_POINT('',#19341);
#5453=VERTEX_POINT('',#19343);
#5454=VERTEX_POINT('',#19347);
#5455=VERTEX_POINT('',#19349);
#5456=VERTEX_POINT('',#19353);
#5457=VERTEX_POINT('',#19355);
#5458=VERTEX_POINT('',#19359);
#5459=VERTEX_POINT('',#19361);
#6625=EDGE_CURVE('',#5317,#5317,#4476,.T.);
#6626=EDGE_CURVE('',#5317,#5318,#2967,.T.);
#6627=EDGE_CURVE('',#5318,#5318,#4477,.T.);
#6628=EDGE_CURVE('',#5319,#5319,#4478,.T.);
#6629=EDGE_CURVE('',#5319,#5320,#2968,.T.);
#6630=EDGE_CURVE('',#5320,#5320,#4479,.T.);
#6631=EDGE_CURVE('',#5321,#5321,#4480,.T.);
#6632=EDGE_CURVE('',#5321,#5322,#2969,.T.);
#6633=EDGE_CURVE('',#5322,#5322,#4481,.T.);
#6634=EDGE_CURVE('',#5323,#5323,#4482,.T.);
#6635=EDGE_CURVE('',#5323,#5324,#2970,.T.);
#6636=EDGE_CURVE('',#5324,#5324,#4483,.T.);
#6637=EDGE_CURVE('',#5325,#5325,#4484,.T.);
#6638=EDGE_CURVE('',#5325,#5326,#2971,.T.);
#6639=EDGE_CURVE('',#5326,#5326,#4485,.T.);
#6640=EDGE_CURVE('',#5327,#5327,#4486,.T.);
#6641=EDGE_CURVE('',#5327,#5328,#2972,.T.);
#6642=EDGE_CURVE('',#5328,#5328,#4487,.T.);
#6643=EDGE_CURVE('',#5329,#5329,#4488,.T.);
#6644=EDGE_CURVE('',#5329,#5330,#2973,.T.);
#6645=EDGE_CURVE('',#5330,#5330,#4489,.T.);
#6646=EDGE_CURVE('',#5331,#5331,#4490,.T.);
#6647=EDGE_CURVE('',#5331,#5332,#2974,.T.);
#6648=EDGE_CURVE('',#5332,#5332,#4491,.T.);
#6649=EDGE_CURVE('',#5333,#5333,#4492,.T.);
#6650=EDGE_CURVE('',#5333,#5334,#2975,.T.);
#6651=EDGE_CURVE('',#5334,#5334,#4493,.T.);
#6652=EDGE_CURVE('',#5335,#5335,#4494,.T.);
#6653=EDGE_CURVE('',#5335,#5336,#2976,.T.);
#6654=EDGE_CURVE('',#5336,#5336,#4495,.T.);
#6655=EDGE_CURVE('',#5337,#5337,#4496,.T.);
#6656=EDGE_CURVE('',#5337,#5338,#2977,.T.);
#6657=EDGE_CURVE('',#5338,#5338,#4497,.T.);
#6658=EDGE_CURVE('',#5339,#5339,#4498,.T.);
#6659=EDGE_CURVE('',#5339,#5340,#2978,.T.);
#6660=EDGE_CURVE('',#5340,#5340,#4499,.T.);
#6661=EDGE_CURVE('',#5341,#5341,#4500,.T.);
#6662=EDGE_CURVE('',#5341,#5342,#2979,.T.);
#6663=EDGE_CURVE('',#5342,#5342,#4501,.T.);
#6664=EDGE_CURVE('',#5343,#5343,#4502,.T.);
#6665=EDGE_CURVE('',#5343,#5344,#2980,.T.);
#6666=EDGE_CURVE('',#5344,#5344,#4503,.T.);
#6667=EDGE_CURVE('',#5345,#5345,#4504,.T.);
#6668=EDGE_CURVE('',#5345,#5346,#2981,.T.);
#6669=EDGE_CURVE('',#5346,#5346,#4505,.T.);
#6670=EDGE_CURVE('',#5347,#5347,#4506,.T.);
#6671=EDGE_CURVE('',#5347,#5348,#2982,.T.);
#6672=EDGE_CURVE('',#5348,#5348,#4507,.T.);
#6673=EDGE_CURVE('',#5349,#5349,#4508,.T.);
#6674=EDGE_CURVE('',#5349,#5350,#2983,.T.);
#6675=EDGE_CURVE('',#5350,#5350,#4509,.T.);
#6676=EDGE_CURVE('',#5351,#5351,#4510,.T.);
#6677=EDGE_CURVE('',#5351,#5352,#2984,.T.);
#6678=EDGE_CURVE('',#5352,#5352,#4511,.T.);
#6679=EDGE_CURVE('',#5353,#5353,#4512,.T.);
#6680=EDGE_CURVE('',#5353,#5354,#2985,.T.);
#6681=EDGE_CURVE('',#5354,#5354,#4513,.T.);
#6682=EDGE_CURVE('',#5355,#5355,#4514,.T.);
#6683=EDGE_CURVE('',#5355,#5356,#2986,.T.);
#6684=EDGE_CURVE('',#5356,#5356,#4515,.T.);
#6685=EDGE_CURVE('',#5357,#5357,#4516,.T.);
#6686=EDGE_CURVE('',#5357,#5358,#2987,.T.);
#6687=EDGE_CURVE('',#5358,#5358,#4517,.T.);
#6688=EDGE_CURVE('',#5359,#5359,#4518,.T.);
#6689=EDGE_CURVE('',#5359,#5360,#2988,.T.);
#6690=EDGE_CURVE('',#5360,#5360,#4519,.T.);
#6691=EDGE_CURVE('',#5361,#5361,#4520,.T.);
#6692=EDGE_CURVE('',#5361,#5362,#2989,.T.);
#6693=EDGE_CURVE('',#5362,#5362,#4521,.T.);
#6694=EDGE_CURVE('',#5363,#5363,#4522,.T.);
#6695=EDGE_CURVE('',#5363,#5364,#2990,.T.);
#6696=EDGE_CURVE('',#5364,#5364,#4523,.T.);
#6697=EDGE_CURVE('',#5365,#5365,#4524,.T.);
#6698=EDGE_CURVE('',#5365,#5366,#2991,.T.);
#6699=EDGE_CURVE('',#5366,#5366,#4525,.T.);
#6700=EDGE_CURVE('',#5326,#5367,#2992,.T.);
#6701=EDGE_CURVE('',#5367,#5367,#4526,.T.);
#6702=EDGE_CURVE('',#5328,#5368,#2993,.T.);
#6703=EDGE_CURVE('',#5368,#5368,#4527,.T.);
#6704=EDGE_CURVE('',#5330,#5369,#2994,.T.);
#6705=EDGE_CURVE('',#5369,#5369,#4528,.T.);
#6706=EDGE_CURVE('',#5332,#5370,#2995,.T.);
#6707=EDGE_CURVE('',#5370,#5370,#4529,.T.);
#6708=EDGE_CURVE('',#5342,#5371,#2996,.T.);
#6709=EDGE_CURVE('',#5371,#5371,#4530,.T.);
#6710=EDGE_CURVE('',#5344,#5372,#2997,.T.);
#6711=EDGE_CURVE('',#5372,#5372,#4531,.T.);
#6712=EDGE_CURVE('',#5346,#5373,#2998,.T.);
#6713=EDGE_CURVE('',#5373,#5373,#4532,.T.);
#6714=EDGE_CURVE('',#5348,#5374,#2999,.T.);
#6715=EDGE_CURVE('',#5374,#5374,#4533,.T.);
#6716=EDGE_CURVE('',#5366,#5375,#3000,.T.);
#6717=EDGE_CURVE('',#5375,#5375,#4534,.T.);
#6718=EDGE_CURVE('',#5376,#5376,#4535,.T.);
#6719=EDGE_CURVE('',#5376,#5377,#3001,.T.);
#6720=EDGE_CURVE('',#5377,#5377,#4536,.T.);
#6721=EDGE_CURVE('',#5378,#5378,#4537,.T.);
#6722=EDGE_CURVE('',#5378,#5379,#3002,.T.);
#6723=EDGE_CURVE('',#5379,#5379,#4538,.T.);
#6724=EDGE_CURVE('',#5380,#5380,#4539,.T.);
#6725=EDGE_CURVE('',#5380,#5381,#3003,.T.);
#6726=EDGE_CURVE('',#5381,#5381,#4540,.T.);
#6727=EDGE_CURVE('',#5382,#5382,#4541,.T.);
#6728=EDGE_CURVE('',#5382,#5383,#3004,.T.);
#6729=EDGE_CURVE('',#5383,#5383,#4542,.T.);
#6730=EDGE_CURVE('',#5384,#5384,#4543,.T.);
#6731=EDGE_CURVE('',#5384,#5385,#3005,.T.);
#6732=EDGE_CURVE('',#5385,#5385,#4544,.T.);
#6733=EDGE_CURVE('',#5386,#5386,#4545,.T.);
#6734=EDGE_CURVE('',#5386,#5387,#3006,.T.);
#6735=EDGE_CURVE('',#5387,#5387,#4546,.T.);
#6736=EDGE_CURVE('',#5388,#5388,#4547,.T.);
#6737=EDGE_CURVE('',#5388,#5389,#3007,.T.);
#6738=EDGE_CURVE('',#5389,#5389,#4548,.T.);
#6739=EDGE_CURVE('',#5390,#5390,#4549,.T.);
#6740=EDGE_CURVE('',#5390,#5391,#3008,.T.);
#6741=EDGE_CURVE('',#5391,#5391,#4550,.T.);
#6742=EDGE_CURVE('',#5392,#5393,#3009,.T.);
#6743=EDGE_CURVE('',#5394,#5392,#3010,.T.);
#6744=EDGE_CURVE('',#5395,#5394,#4551,.T.);
#6745=EDGE_CURVE('',#5396,#5395,#3011,.T.);
#6746=EDGE_CURVE('',#5397,#5396,#4552,.T.);
#6747=EDGE_CURVE('',#5393,#5397,#3012,.T.);
#6748=EDGE_CURVE('',#5398,#5393,#4553,.T.);
#6749=EDGE_CURVE('',#5399,#5397,#288,.T.);
#6750=EDGE_CURVE('',#5399,#5400,#203,.T.);
#6751=EDGE_CURVE('',#5398,#5400,#3013,.T.);
#6752=EDGE_CURVE('',#5398,#5401,#3014,.T.);
#6753=EDGE_CURVE('',#5402,#5401,#3015,.T.);
#6754=EDGE_CURVE('',#5403,#5402,#3016,.T.);
#6755=EDGE_CURVE('',#5404,#5403,#4554,.T.);
#6756=EDGE_CURVE('',#5405,#5404,#3017,.T.);
#6757=EDGE_CURVE('',#5406,#5405,#4555,.T.);
#6758=EDGE_CURVE('',#5407,#5406,#3018,.T.);
#6759=EDGE_CURVE('',#5408,#5407,#3019,.T.);
#6760=EDGE_CURVE('',#5408,#5409,#3020,.T.);
#6761=EDGE_CURVE('',#5409,#5392,#4556,.T.);
#6762=EDGE_CURVE('',#5410,#5409,#3021,.T.);
#6763=EDGE_CURVE('',#5411,#5410,#204,.T.);
#6764=EDGE_CURVE('',#5394,#5411,#289,.T.);
#6765=EDGE_CURVE('',#5412,#5394,#3022,.T.);
#6766=EDGE_CURVE('',#5413,#5412,#3023,.T.);
#6767=EDGE_CURVE('',#5414,#5413,#4557,.T.);
#6768=EDGE_CURVE('',#5395,#5414,#3024,.T.);
#6769=EDGE_CURVE('',#5414,#5415,#3025,.T.);
#6770=EDGE_CURVE('',#5415,#5396,#3026,.T.);
#6771=EDGE_CURVE('',#5416,#5415,#4558,.T.);
#6772=EDGE_CURVE('',#5417,#5416,#3027,.T.);
#6773=EDGE_CURVE('',#5397,#5417,#3028,.T.);
#6774=EDGE_CURVE('',#5404,#5416,#3029,.T.);
#6775=EDGE_CURVE('',#5413,#5405,#3030,.T.);
#6776=EDGE_CURVE('',#5418,#5400,#3031,.T.);
#6777=EDGE_CURVE('',#5419,#5418,#4559,.T.);
#6778=EDGE_CURVE('',#5420,#5419,#3032,.T.);
#6779=EDGE_CURVE('',#5421,#5420,#4560,.T.);
#6780=EDGE_CURVE('',#5422,#5421,#3033,.T.);
#6781=EDGE_CURVE('',#5401,#5422,#4561,.T.);
#6782=EDGE_CURVE('',#5423,#5416,#290,.T.);
#6783=EDGE_CURVE('',#5399,#5423,#3034,.T.);
#6784=EDGE_CURVE('',#5424,#5411,#3035,.T.);
#6785=EDGE_CURVE('',#5413,#5424,#291,.T.);
#6786=EDGE_CURVE('',#5425,#5426,#4562,.T.);
#6787=EDGE_CURVE('',#5427,#5425,#3036,.T.);
#6788=EDGE_CURVE('',#5428,#5427,#4563,.T.);
#6789=EDGE_CURVE('',#5410,#5428,#3037,.T.);
#6790=EDGE_CURVE('',#5429,#5408,#4564,.T.);
#6791=EDGE_CURVE('',#5426,#5429,#3038,.T.);
#6792=EDGE_CURVE('',#5403,#5430,#3039,.T.);
#6793=EDGE_CURVE('',#5430,#5423,#4565,.T.);
#6794=EDGE_CURVE('',#5424,#5431,#4566,.T.);
#6795=EDGE_CURVE('',#5431,#5406,#3040,.T.);
#6796=EDGE_CURVE('',#5430,#5432,#3041,.T.);
#6797=EDGE_CURVE('',#5432,#5418,#3042,.T.);
#6798=EDGE_CURVE('',#5400,#5433,#3043,.T.);
#6799=EDGE_CURVE('',#5433,#5430,#3044,.T.);
#6800=EDGE_CURVE('',#5432,#5434,#4567,.T.);
#6801=EDGE_CURVE('',#5434,#5419,#3045,.T.);
#6802=EDGE_CURVE('',#5420,#5435,#3046,.T.);
#6803=EDGE_CURVE('',#5435,#5436,#4568,.T.);
#6804=EDGE_CURVE('',#5436,#5421,#3047,.T.);
#6805=EDGE_CURVE('',#5436,#5437,#3048,.T.);
#6806=EDGE_CURVE('',#5437,#5422,#3049,.T.);
#6807=EDGE_CURVE('',#5437,#5402,#4569,.T.);
#6808=EDGE_CURVE('',#5410,#5438,#3050,.T.);
#6809=EDGE_CURVE('',#5438,#5431,#3051,.T.);
#6810=EDGE_CURVE('',#5426,#5439,#3052,.T.);
#6811=EDGE_CURVE('',#5440,#5429,#3053,.T.);
#6812=EDGE_CURVE('',#5439,#5440,#3054,.T.);
#6813=EDGE_CURVE('',#5439,#5441,#4570,.T.);
#6814=EDGE_CURVE('',#5441,#5425,#3055,.T.);
#6815=EDGE_CURVE('',#5427,#5442,#3056,.T.);
#6816=EDGE_CURVE('',#5442,#5443,#4571,.T.);
#6817=EDGE_CURVE('',#5443,#5428,#3057,.T.);
#6818=EDGE_CURVE('',#5443,#5431,#3058,.T.);
#6819=EDGE_CURVE('',#5407,#5440,#4572,.T.);
#6820=EDGE_CURVE('',#5435,#5434,#3059,.T.);
#6821=EDGE_CURVE('',#5442,#5441,#3060,.T.);
#6822=EDGE_CURVE('',#5444,#5444,#4573,.T.);
#6823=EDGE_CURVE('',#5444,#5445,#3061,.T.);
#6824=EDGE_CURVE('',#5445,#5445,#4574,.T.);
#6825=EDGE_CURVE('',#5446,#5446,#4575,.T.);
#6826=EDGE_CURVE('',#5446,#5447,#3062,.T.);
#6827=EDGE_CURVE('',#5447,#5447,#4576,.T.);
#6828=EDGE_CURVE('',#5448,#5448,#4577,.T.);
#6829=EDGE_CURVE('',#5448,#5449,#3063,.T.);
#6830=EDGE_CURVE('',#5449,#5449,#4578,.T.);
#6831=EDGE_CURVE('',#5450,#5450,#4579,.T.);
#6832=EDGE_CURVE('',#5450,#5451,#3064,.T.);
#6833=EDGE_CURVE('',#5451,#5451,#4580,.T.);
#6834=EDGE_CURVE('',#5452,#5452,#4581,.T.);
#6835=EDGE_CURVE('',#5452,#5453,#3065,.T.);
#6836=EDGE_CURVE('',#5453,#5453,#4582,.T.);
#6837=EDGE_CURVE('',#5454,#5454,#4583,.T.);
#6838=EDGE_CURVE('',#5454,#5455,#3066,.T.);
#6839=EDGE_CURVE('',#5455,#5455,#4584,.T.);
#6840=EDGE_CURVE('',#5456,#5456,#4585,.T.);
#6841=EDGE_CURVE('',#5456,#5457,#3067,.T.);
#6842=EDGE_CURVE('',#5457,#5457,#4586,.T.);
#6843=EDGE_CURVE('',#5458,#5458,#4587,.T.);
#6844=EDGE_CURVE('',#5458,#5459,#3068,.T.);
#6845=EDGE_CURVE('',#5459,#5459,#4588,.T.);
#9045=ORIENTED_EDGE('',*,*,#6625,.F.);
#9046=ORIENTED_EDGE('',*,*,#6626,.T.);
#9047=ORIENTED_EDGE('',*,*,#6627,.T.);
#9048=ORIENTED_EDGE('',*,*,#6626,.F.);
#9049=ORIENTED_EDGE('',*,*,#6628,.F.);
#9050=ORIENTED_EDGE('',*,*,#6629,.T.);
#9051=ORIENTED_EDGE('',*,*,#6630,.T.);
#9052=ORIENTED_EDGE('',*,*,#6629,.F.);
#9053=ORIENTED_EDGE('',*,*,#6631,.F.);
#9054=ORIENTED_EDGE('',*,*,#6632,.T.);
#9055=ORIENTED_EDGE('',*,*,#6633,.T.);
#9056=ORIENTED_EDGE('',*,*,#6632,.F.);
#9057=ORIENTED_EDGE('',*,*,#6634,.F.);
#9058=ORIENTED_EDGE('',*,*,#6635,.T.);
#9059=ORIENTED_EDGE('',*,*,#6636,.T.);
#9060=ORIENTED_EDGE('',*,*,#6635,.F.);
#9061=ORIENTED_EDGE('',*,*,#6637,.T.);
#9062=ORIENTED_EDGE('',*,*,#6638,.T.);
#9063=ORIENTED_EDGE('',*,*,#6639,.F.);
#9064=ORIENTED_EDGE('',*,*,#6638,.F.);
#9065=ORIENTED_EDGE('',*,*,#6640,.T.);
#9066=ORIENTED_EDGE('',*,*,#6641,.T.);
#9067=ORIENTED_EDGE('',*,*,#6642,.F.);
#9068=ORIENTED_EDGE('',*,*,#6641,.F.);
#9069=ORIENTED_EDGE('',*,*,#6643,.T.);
#9070=ORIENTED_EDGE('',*,*,#6644,.T.);
#9071=ORIENTED_EDGE('',*,*,#6645,.F.);
#9072=ORIENTED_EDGE('',*,*,#6644,.F.);
#9073=ORIENTED_EDGE('',*,*,#6646,.T.);
#9074=ORIENTED_EDGE('',*,*,#6647,.T.);
#9075=ORIENTED_EDGE('',*,*,#6648,.F.);
#9076=ORIENTED_EDGE('',*,*,#6647,.F.);
#9077=ORIENTED_EDGE('',*,*,#6649,.F.);
#9078=ORIENTED_EDGE('',*,*,#6650,.T.);
#9079=ORIENTED_EDGE('',*,*,#6651,.T.);
#9080=ORIENTED_EDGE('',*,*,#6650,.F.);
#9081=ORIENTED_EDGE('',*,*,#6652,.F.);
#9082=ORIENTED_EDGE('',*,*,#6653,.T.);
#9083=ORIENTED_EDGE('',*,*,#6654,.T.);
#9084=ORIENTED_EDGE('',*,*,#6653,.F.);
#9085=ORIENTED_EDGE('',*,*,#6655,.F.);
#9086=ORIENTED_EDGE('',*,*,#6656,.T.);
#9087=ORIENTED_EDGE('',*,*,#6657,.T.);
#9088=ORIENTED_EDGE('',*,*,#6656,.F.);
#9089=ORIENTED_EDGE('',*,*,#6658,.F.);
#9090=ORIENTED_EDGE('',*,*,#6659,.T.);
#9091=ORIENTED_EDGE('',*,*,#6660,.T.);
#9092=ORIENTED_EDGE('',*,*,#6659,.F.);
#9093=ORIENTED_EDGE('',*,*,#6661,.T.);
#9094=ORIENTED_EDGE('',*,*,#6662,.T.);
#9095=ORIENTED_EDGE('',*,*,#6663,.F.);
#9096=ORIENTED_EDGE('',*,*,#6662,.F.);
#9097=ORIENTED_EDGE('',*,*,#6664,.T.);
#9098=ORIENTED_EDGE('',*,*,#6665,.T.);
#9099=ORIENTED_EDGE('',*,*,#6666,.F.);
#9100=ORIENTED_EDGE('',*,*,#6665,.F.);
#9101=ORIENTED_EDGE('',*,*,#6667,.T.);
#9102=ORIENTED_EDGE('',*,*,#6668,.T.);
#9103=ORIENTED_EDGE('',*,*,#6669,.F.);
#9104=ORIENTED_EDGE('',*,*,#6668,.F.);
#9105=ORIENTED_EDGE('',*,*,#6670,.T.);
#9106=ORIENTED_EDGE('',*,*,#6671,.T.);
#9107=ORIENTED_EDGE('',*,*,#6672,.F.);
#9108=ORIENTED_EDGE('',*,*,#6671,.F.);
#9109=ORIENTED_EDGE('',*,*,#6673,.T.);
#9110=ORIENTED_EDGE('',*,*,#6674,.T.);
#9111=ORIENTED_EDGE('',*,*,#6675,.F.);
#9112=ORIENTED_EDGE('',*,*,#6674,.F.);
#9113=ORIENTED_EDGE('',*,*,#6676,.T.);
#9114=ORIENTED_EDGE('',*,*,#6677,.T.);
#9115=ORIENTED_EDGE('',*,*,#6678,.F.);
#9116=ORIENTED_EDGE('',*,*,#6677,.F.);
#9117=ORIENTED_EDGE('',*,*,#6679,.T.);
#9118=ORIENTED_EDGE('',*,*,#6680,.T.);
#9119=ORIENTED_EDGE('',*,*,#6681,.F.);
#9120=ORIENTED_EDGE('',*,*,#6680,.F.);
#9121=ORIENTED_EDGE('',*,*,#6682,.T.);
#9122=ORIENTED_EDGE('',*,*,#6683,.T.);
#9123=ORIENTED_EDGE('',*,*,#6684,.F.);
#9124=ORIENTED_EDGE('',*,*,#6683,.F.);
#9125=ORIENTED_EDGE('',*,*,#6685,.T.);
#9126=ORIENTED_EDGE('',*,*,#6686,.T.);
#9127=ORIENTED_EDGE('',*,*,#6687,.F.);
#9128=ORIENTED_EDGE('',*,*,#6686,.F.);
#9129=ORIENTED_EDGE('',*,*,#6688,.T.);
#9130=ORIENTED_EDGE('',*,*,#6689,.T.);
#9131=ORIENTED_EDGE('',*,*,#6690,.F.);
#9132=ORIENTED_EDGE('',*,*,#6689,.F.);
#9133=ORIENTED_EDGE('',*,*,#6691,.T.);
#9134=ORIENTED_EDGE('',*,*,#6692,.T.);
#9135=ORIENTED_EDGE('',*,*,#6693,.F.);
#9136=ORIENTED_EDGE('',*,*,#6692,.F.);
#9137=ORIENTED_EDGE('',*,*,#6694,.T.);
#9138=ORIENTED_EDGE('',*,*,#6695,.T.);
#9139=ORIENTED_EDGE('',*,*,#6696,.F.);
#9140=ORIENTED_EDGE('',*,*,#6695,.F.);
#9141=ORIENTED_EDGE('',*,*,#6697,.T.);
#9142=ORIENTED_EDGE('',*,*,#6698,.T.);
#9143=ORIENTED_EDGE('',*,*,#6699,.F.);
#9144=ORIENTED_EDGE('',*,*,#6698,.F.);
#9145=ORIENTED_EDGE('',*,*,#6639,.T.);
#9146=ORIENTED_EDGE('',*,*,#6700,.T.);
#9147=ORIENTED_EDGE('',*,*,#6701,.F.);
#9148=ORIENTED_EDGE('',*,*,#6700,.F.);
#9149=ORIENTED_EDGE('',*,*,#6642,.T.);
#9150=ORIENTED_EDGE('',*,*,#6702,.T.);
#9151=ORIENTED_EDGE('',*,*,#6703,.F.);
#9152=ORIENTED_EDGE('',*,*,#6702,.F.);
#9153=ORIENTED_EDGE('',*,*,#6645,.T.);
#9154=ORIENTED_EDGE('',*,*,#6704,.T.);
#9155=ORIENTED_EDGE('',*,*,#6705,.F.);
#9156=ORIENTED_EDGE('',*,*,#6704,.F.);
#9157=ORIENTED_EDGE('',*,*,#6648,.T.);
#9158=ORIENTED_EDGE('',*,*,#6706,.T.);
#9159=ORIENTED_EDGE('',*,*,#6707,.F.);
#9160=ORIENTED_EDGE('',*,*,#6706,.F.);
#9161=ORIENTED_EDGE('',*,*,#6663,.T.);
#9162=ORIENTED_EDGE('',*,*,#6708,.T.);
#9163=ORIENTED_EDGE('',*,*,#6709,.F.);
#9164=ORIENTED_EDGE('',*,*,#6708,.F.);
#9165=ORIENTED_EDGE('',*,*,#6666,.T.);
#9166=ORIENTED_EDGE('',*,*,#6710,.T.);
#9167=ORIENTED_EDGE('',*,*,#6711,.F.);
#9168=ORIENTED_EDGE('',*,*,#6710,.F.);
#9169=ORIENTED_EDGE('',*,*,#6669,.T.);
#9170=ORIENTED_EDGE('',*,*,#6712,.T.);
#9171=ORIENTED_EDGE('',*,*,#6713,.F.);
#9172=ORIENTED_EDGE('',*,*,#6712,.F.);
#9173=ORIENTED_EDGE('',*,*,#6672,.T.);
#9174=ORIENTED_EDGE('',*,*,#6714,.T.);
#9175=ORIENTED_EDGE('',*,*,#6715,.F.);
#9176=ORIENTED_EDGE('',*,*,#6714,.F.);
#9177=ORIENTED_EDGE('',*,*,#6699,.T.);
#9178=ORIENTED_EDGE('',*,*,#6716,.T.);
#9179=ORIENTED_EDGE('',*,*,#6717,.F.);
#9180=ORIENTED_EDGE('',*,*,#6716,.F.);
#9181=ORIENTED_EDGE('',*,*,#6718,.F.);
#9182=ORIENTED_EDGE('',*,*,#6719,.T.);
#9183=ORIENTED_EDGE('',*,*,#6720,.T.);
#9184=ORIENTED_EDGE('',*,*,#6719,.F.);
#9185=ORIENTED_EDGE('',*,*,#6721,.F.);
#9186=ORIENTED_EDGE('',*,*,#6722,.T.);
#9187=ORIENTED_EDGE('',*,*,#6723,.T.);
#9188=ORIENTED_EDGE('',*,*,#6722,.F.);
#9189=ORIENTED_EDGE('',*,*,#6724,.F.);
#9190=ORIENTED_EDGE('',*,*,#6725,.T.);
#9191=ORIENTED_EDGE('',*,*,#6726,.T.);
#9192=ORIENTED_EDGE('',*,*,#6725,.F.);
#9193=ORIENTED_EDGE('',*,*,#6727,.F.);
#9194=ORIENTED_EDGE('',*,*,#6728,.T.);
#9195=ORIENTED_EDGE('',*,*,#6729,.T.);
#9196=ORIENTED_EDGE('',*,*,#6728,.F.);
#9197=ORIENTED_EDGE('',*,*,#6730,.T.);
#9198=ORIENTED_EDGE('',*,*,#6731,.T.);
#9199=ORIENTED_EDGE('',*,*,#6732,.F.);
#9200=ORIENTED_EDGE('',*,*,#6731,.F.);
#9201=ORIENTED_EDGE('',*,*,#6733,.T.);
#9202=ORIENTED_EDGE('',*,*,#6734,.T.);
#9203=ORIENTED_EDGE('',*,*,#6735,.F.);
#9204=ORIENTED_EDGE('',*,*,#6734,.F.);
#9205=ORIENTED_EDGE('',*,*,#6736,.T.);
#9206=ORIENTED_EDGE('',*,*,#6737,.T.);
#9207=ORIENTED_EDGE('',*,*,#6738,.F.);
#9208=ORIENTED_EDGE('',*,*,#6737,.F.);
#9209=ORIENTED_EDGE('',*,*,#6739,.T.);
#9210=ORIENTED_EDGE('',*,*,#6740,.T.);
#9211=ORIENTED_EDGE('',*,*,#6741,.F.);
#9212=ORIENTED_EDGE('',*,*,#6740,.F.);
#9213=ORIENTED_EDGE('',*,*,#6742,.F.);
#9214=ORIENTED_EDGE('',*,*,#6743,.F.);
#9215=ORIENTED_EDGE('',*,*,#6744,.F.);
#9216=ORIENTED_EDGE('',*,*,#6745,.F.);
#9217=ORIENTED_EDGE('',*,*,#6746,.F.);
#9218=ORIENTED_EDGE('',*,*,#6747,.F.);
#9219=ORIENTED_EDGE('',*,*,#6627,.F.);
#9220=ORIENTED_EDGE('',*,*,#6630,.F.);
#9221=ORIENTED_EDGE('',*,*,#6633,.F.);
#9222=ORIENTED_EDGE('',*,*,#6636,.F.);
#9223=ORIENTED_EDGE('',*,*,#6637,.F.);
#9224=ORIENTED_EDGE('',*,*,#6640,.F.);
#9225=ORIENTED_EDGE('',*,*,#6643,.F.);
#9226=ORIENTED_EDGE('',*,*,#6646,.F.);
#9227=ORIENTED_EDGE('',*,*,#6651,.F.);
#9228=ORIENTED_EDGE('',*,*,#6654,.F.);
#9229=ORIENTED_EDGE('',*,*,#6657,.F.);
#9230=ORIENTED_EDGE('',*,*,#6660,.F.);
#9231=ORIENTED_EDGE('',*,*,#6661,.F.);
#9232=ORIENTED_EDGE('',*,*,#6664,.F.);
#9233=ORIENTED_EDGE('',*,*,#6667,.F.);
#9234=ORIENTED_EDGE('',*,*,#6670,.F.);
#9235=ORIENTED_EDGE('',*,*,#6673,.F.);
#9236=ORIENTED_EDGE('',*,*,#6676,.F.);
#9237=ORIENTED_EDGE('',*,*,#6679,.F.);
#9238=ORIENTED_EDGE('',*,*,#6682,.F.);
#9239=ORIENTED_EDGE('',*,*,#6685,.F.);
#9240=ORIENTED_EDGE('',*,*,#6688,.F.);
#9241=ORIENTED_EDGE('',*,*,#6691,.F.);
#9242=ORIENTED_EDGE('',*,*,#6694,.F.);
#9243=ORIENTED_EDGE('',*,*,#6697,.F.);
#9244=ORIENTED_EDGE('',*,*,#6748,.T.);
#9245=ORIENTED_EDGE('',*,*,#6747,.T.);
#9246=ORIENTED_EDGE('',*,*,#6749,.F.);
#9247=ORIENTED_EDGE('',*,*,#6750,.T.);
#9248=ORIENTED_EDGE('',*,*,#6751,.F.);
#9249=ORIENTED_EDGE('',*,*,#6742,.T.);
#9250=ORIENTED_EDGE('',*,*,#6748,.F.);
#9251=ORIENTED_EDGE('',*,*,#6752,.T.);
#9252=ORIENTED_EDGE('',*,*,#6753,.F.);
#9253=ORIENTED_EDGE('',*,*,#6754,.F.);
#9254=ORIENTED_EDGE('',*,*,#6755,.F.);
#9255=ORIENTED_EDGE('',*,*,#6756,.F.);
#9256=ORIENTED_EDGE('',*,*,#6757,.F.);
#9257=ORIENTED_EDGE('',*,*,#6758,.F.);
#9258=ORIENTED_EDGE('',*,*,#6759,.F.);
#9259=ORIENTED_EDGE('',*,*,#6760,.T.);
#9260=ORIENTED_EDGE('',*,*,#6761,.T.);
#9261=ORIENTED_EDGE('',*,*,#6743,.T.);
#9262=ORIENTED_EDGE('',*,*,#6761,.F.);
#9263=ORIENTED_EDGE('',*,*,#6762,.F.);
#9264=ORIENTED_EDGE('',*,*,#6763,.F.);
#9265=ORIENTED_EDGE('',*,*,#6764,.F.);
#9266=ORIENTED_EDGE('',*,*,#6744,.T.);
#9267=ORIENTED_EDGE('',*,*,#6765,.F.);
#9268=ORIENTED_EDGE('',*,*,#6766,.F.);
#9269=ORIENTED_EDGE('',*,*,#6767,.F.);
#9270=ORIENTED_EDGE('',*,*,#6768,.F.);
#9271=ORIENTED_EDGE('',*,*,#6768,.T.);
#9272=ORIENTED_EDGE('',*,*,#6769,.T.);
#9273=ORIENTED_EDGE('',*,*,#6770,.T.);
#9274=ORIENTED_EDGE('',*,*,#6745,.T.);
#9275=ORIENTED_EDGE('',*,*,#6746,.T.);
#9276=ORIENTED_EDGE('',*,*,#6770,.F.);
#9277=ORIENTED_EDGE('',*,*,#6771,.F.);
#9278=ORIENTED_EDGE('',*,*,#6772,.F.);
#9279=ORIENTED_EDGE('',*,*,#6773,.F.);
#9280=ORIENTED_EDGE('',*,*,#6774,.T.);
#9281=ORIENTED_EDGE('',*,*,#6771,.T.);
#9282=ORIENTED_EDGE('',*,*,#6769,.F.);
#9283=ORIENTED_EDGE('',*,*,#6767,.T.);
#9284=ORIENTED_EDGE('',*,*,#6775,.T.);
#9285=ORIENTED_EDGE('',*,*,#6756,.T.);
#9286=ORIENTED_EDGE('',*,*,#6625,.T.);
#9287=ORIENTED_EDGE('',*,*,#6628,.T.);
#9288=ORIENTED_EDGE('',*,*,#6631,.T.);
#9289=ORIENTED_EDGE('',*,*,#6634,.T.);
#9290=ORIENTED_EDGE('',*,*,#6701,.T.);
#9291=ORIENTED_EDGE('',*,*,#6703,.T.);
#9292=ORIENTED_EDGE('',*,*,#6705,.T.);
#9293=ORIENTED_EDGE('',*,*,#6707,.T.);
#9294=ORIENTED_EDGE('',*,*,#6649,.T.);
#9295=ORIENTED_EDGE('',*,*,#6652,.T.);
#9296=ORIENTED_EDGE('',*,*,#6655,.T.);
#9297=ORIENTED_EDGE('',*,*,#6658,.T.);
#9298=ORIENTED_EDGE('',*,*,#6709,.T.);
#9299=ORIENTED_EDGE('',*,*,#6711,.T.);
#9300=ORIENTED_EDGE('',*,*,#6713,.T.);
#9301=ORIENTED_EDGE('',*,*,#6715,.T.);
#9302=ORIENTED_EDGE('',*,*,#6717,.T.);
#9303=ORIENTED_EDGE('',*,*,#6675,.T.);
#9304=ORIENTED_EDGE('',*,*,#6678,.T.);
#9305=ORIENTED_EDGE('',*,*,#6681,.T.);
#9306=ORIENTED_EDGE('',*,*,#6684,.T.);
#9307=ORIENTED_EDGE('',*,*,#6687,.T.);
#9308=ORIENTED_EDGE('',*,*,#6690,.T.);
#9309=ORIENTED_EDGE('',*,*,#6693,.T.);
#9310=ORIENTED_EDGE('',*,*,#6696,.T.);
#9311=ORIENTED_EDGE('',*,*,#6751,.T.);
#9312=ORIENTED_EDGE('',*,*,#6776,.F.);
#9313=ORIENTED_EDGE('',*,*,#6777,.F.);
#9314=ORIENTED_EDGE('',*,*,#6778,.F.);
#9315=ORIENTED_EDGE('',*,*,#6779,.F.);
#9316=ORIENTED_EDGE('',*,*,#6780,.F.);
#9317=ORIENTED_EDGE('',*,*,#6781,.F.);
#9318=ORIENTED_EDGE('',*,*,#6752,.F.);
#9319=ORIENTED_EDGE('',*,*,#6720,.F.);
#9320=ORIENTED_EDGE('',*,*,#6723,.F.);
#9321=ORIENTED_EDGE('',*,*,#6726,.F.);
#9322=ORIENTED_EDGE('',*,*,#6729,.F.);
#9323=ORIENTED_EDGE('',*,*,#6749,.T.);
#9324=ORIENTED_EDGE('',*,*,#6773,.T.);
#9325=ORIENTED_EDGE('',*,*,#6772,.T.);
#9326=ORIENTED_EDGE('',*,*,#6782,.F.);
#9327=ORIENTED_EDGE('',*,*,#6783,.F.);
#9328=ORIENTED_EDGE('',*,*,#6764,.T.);
#9329=ORIENTED_EDGE('',*,*,#6784,.F.);
#9330=ORIENTED_EDGE('',*,*,#6785,.F.);
#9331=ORIENTED_EDGE('',*,*,#6766,.T.);
#9332=ORIENTED_EDGE('',*,*,#6765,.T.);
#9333=ORIENTED_EDGE('',*,*,#6786,.F.);
#9334=ORIENTED_EDGE('',*,*,#6787,.F.);
#9335=ORIENTED_EDGE('',*,*,#6788,.F.);
#9336=ORIENTED_EDGE('',*,*,#6789,.F.);
#9337=ORIENTED_EDGE('',*,*,#6762,.T.);
#9338=ORIENTED_EDGE('',*,*,#6760,.F.);
#9339=ORIENTED_EDGE('',*,*,#6790,.F.);
#9340=ORIENTED_EDGE('',*,*,#6791,.F.);
#9341=ORIENTED_EDGE('',*,*,#6730,.F.);
#9342=ORIENTED_EDGE('',*,*,#6733,.F.);
#9343=ORIENTED_EDGE('',*,*,#6736,.F.);
#9344=ORIENTED_EDGE('',*,*,#6739,.F.);
#9345=ORIENTED_EDGE('',*,*,#6792,.T.);
#9346=ORIENTED_EDGE('',*,*,#6793,.T.);
#9347=ORIENTED_EDGE('',*,*,#6782,.T.);
#9348=ORIENTED_EDGE('',*,*,#6774,.F.);
#9349=ORIENTED_EDGE('',*,*,#6755,.T.);
#9350=ORIENTED_EDGE('',*,*,#6785,.T.);
#9351=ORIENTED_EDGE('',*,*,#6794,.T.);
#9352=ORIENTED_EDGE('',*,*,#6795,.T.);
#9353=ORIENTED_EDGE('',*,*,#6757,.T.);
#9354=ORIENTED_EDGE('',*,*,#6775,.F.);
#9355=ORIENTED_EDGE('',*,*,#6796,.T.);
#9356=ORIENTED_EDGE('',*,*,#6797,.T.);
#9357=ORIENTED_EDGE('',*,*,#6776,.T.);
#9358=ORIENTED_EDGE('',*,*,#6798,.T.);
#9359=ORIENTED_EDGE('',*,*,#6799,.T.);
#9360=ORIENTED_EDGE('',*,*,#6797,.F.);
#9361=ORIENTED_EDGE('',*,*,#6800,.T.);
#9362=ORIENTED_EDGE('',*,*,#6801,.T.);
#9363=ORIENTED_EDGE('',*,*,#6777,.T.);
#9364=ORIENTED_EDGE('',*,*,#6802,.T.);
#9365=ORIENTED_EDGE('',*,*,#6803,.T.);
#9366=ORIENTED_EDGE('',*,*,#6804,.T.);
#9367=ORIENTED_EDGE('',*,*,#6779,.T.);
#9368=ORIENTED_EDGE('',*,*,#6805,.T.);
#9369=ORIENTED_EDGE('',*,*,#6806,.T.);
#9370=ORIENTED_EDGE('',*,*,#6780,.T.);
#9371=ORIENTED_EDGE('',*,*,#6804,.F.);
#9372=ORIENTED_EDGE('',*,*,#6806,.F.);
#9373=ORIENTED_EDGE('',*,*,#6807,.T.);
#9374=ORIENTED_EDGE('',*,*,#6753,.T.);
#9375=ORIENTED_EDGE('',*,*,#6781,.T.);
#9376=ORIENTED_EDGE('',*,*,#6750,.F.);
#9377=ORIENTED_EDGE('',*,*,#6783,.T.);
#9378=ORIENTED_EDGE('',*,*,#6793,.F.);
#9379=ORIENTED_EDGE('',*,*,#6799,.F.);
#9380=ORIENTED_EDGE('',*,*,#6798,.F.);
#9381=ORIENTED_EDGE('',*,*,#6808,.T.);
#9382=ORIENTED_EDGE('',*,*,#6809,.T.);
#9383=ORIENTED_EDGE('',*,*,#6794,.F.);
#9384=ORIENTED_EDGE('',*,*,#6784,.T.);
#9385=ORIENTED_EDGE('',*,*,#6763,.T.);
#9386=ORIENTED_EDGE('',*,*,#6810,.F.);
#9387=ORIENTED_EDGE('',*,*,#6791,.T.);
#9388=ORIENTED_EDGE('',*,*,#6811,.F.);
#9389=ORIENTED_EDGE('',*,*,#6812,.F.);
#9390=ORIENTED_EDGE('',*,*,#6810,.T.);
#9391=ORIENTED_EDGE('',*,*,#6813,.T.);
#9392=ORIENTED_EDGE('',*,*,#6814,.T.);
#9393=ORIENTED_EDGE('',*,*,#6786,.T.);
#9394=ORIENTED_EDGE('',*,*,#6815,.T.);
#9395=ORIENTED_EDGE('',*,*,#6816,.T.);
#9396=ORIENTED_EDGE('',*,*,#6817,.T.);
#9397=ORIENTED_EDGE('',*,*,#6788,.T.);
#9398=ORIENTED_EDGE('',*,*,#6789,.T.);
#9399=ORIENTED_EDGE('',*,*,#6817,.F.);
#9400=ORIENTED_EDGE('',*,*,#6818,.T.);
#9401=ORIENTED_EDGE('',*,*,#6809,.F.);
#9402=ORIENTED_EDGE('',*,*,#6808,.F.);
#9403=ORIENTED_EDGE('',*,*,#6759,.T.);
#9404=ORIENTED_EDGE('',*,*,#6819,.T.);
#9405=ORIENTED_EDGE('',*,*,#6811,.T.);
#9406=ORIENTED_EDGE('',*,*,#6790,.T.);
#9407=ORIENTED_EDGE('',*,*,#6754,.T.);
#9408=ORIENTED_EDGE('',*,*,#6807,.F.);
#9409=ORIENTED_EDGE('',*,*,#6805,.F.);
#9410=ORIENTED_EDGE('',*,*,#6803,.F.);
#9411=ORIENTED_EDGE('',*,*,#6820,.T.);
#9412=ORIENTED_EDGE('',*,*,#6800,.F.);
#9413=ORIENTED_EDGE('',*,*,#6796,.F.);
#9414=ORIENTED_EDGE('',*,*,#6792,.F.);
#9415=ORIENTED_EDGE('',*,*,#6718,.T.);
#9416=ORIENTED_EDGE('',*,*,#6721,.T.);
#9417=ORIENTED_EDGE('',*,*,#6724,.T.);
#9418=ORIENTED_EDGE('',*,*,#6727,.T.);
#9419=ORIENTED_EDGE('',*,*,#6812,.T.);
#9420=ORIENTED_EDGE('',*,*,#6819,.F.);
#9421=ORIENTED_EDGE('',*,*,#6758,.T.);
#9422=ORIENTED_EDGE('',*,*,#6795,.F.);
#9423=ORIENTED_EDGE('',*,*,#6818,.F.);
#9424=ORIENTED_EDGE('',*,*,#6816,.F.);
#9425=ORIENTED_EDGE('',*,*,#6821,.T.);
#9426=ORIENTED_EDGE('',*,*,#6813,.F.);
#9427=ORIENTED_EDGE('',*,*,#6732,.T.);
#9428=ORIENTED_EDGE('',*,*,#6735,.T.);
#9429=ORIENTED_EDGE('',*,*,#6738,.T.);
#9430=ORIENTED_EDGE('',*,*,#6741,.T.);
#9431=ORIENTED_EDGE('',*,*,#6820,.F.);
#9432=ORIENTED_EDGE('',*,*,#6802,.F.);
#9433=ORIENTED_EDGE('',*,*,#6778,.T.);
#9434=ORIENTED_EDGE('',*,*,#6801,.F.);
#9435=ORIENTED_EDGE('',*,*,#6787,.T.);
#9436=ORIENTED_EDGE('',*,*,#6814,.F.);
#9437=ORIENTED_EDGE('',*,*,#6821,.F.);
#9438=ORIENTED_EDGE('',*,*,#6815,.F.);
#9439=ORIENTED_EDGE('',*,*,#6822,.T.);
#9440=ORIENTED_EDGE('',*,*,#6823,.T.);
#9441=ORIENTED_EDGE('',*,*,#6824,.T.);
#9442=ORIENTED_EDGE('',*,*,#6823,.F.);
#9443=ORIENTED_EDGE('',*,*,#6825,.T.);
#9444=ORIENTED_EDGE('',*,*,#6826,.T.);
#9445=ORIENTED_EDGE('',*,*,#6827,.T.);
#9446=ORIENTED_EDGE('',*,*,#6826,.F.);
#9447=ORIENTED_EDGE('',*,*,#6828,.T.);
#9448=ORIENTED_EDGE('',*,*,#6829,.T.);
#9449=ORIENTED_EDGE('',*,*,#6830,.T.);
#9450=ORIENTED_EDGE('',*,*,#6829,.F.);
#9451=ORIENTED_EDGE('',*,*,#6831,.T.);
#9452=ORIENTED_EDGE('',*,*,#6832,.T.);
#9453=ORIENTED_EDGE('',*,*,#6833,.T.);
#9454=ORIENTED_EDGE('',*,*,#6832,.F.);
#9455=ORIENTED_EDGE('',*,*,#6834,.T.);
#9456=ORIENTED_EDGE('',*,*,#6835,.T.);
#9457=ORIENTED_EDGE('',*,*,#6836,.T.);
#9458=ORIENTED_EDGE('',*,*,#6835,.F.);
#9459=ORIENTED_EDGE('',*,*,#6837,.T.);
#9460=ORIENTED_EDGE('',*,*,#6838,.T.);
#9461=ORIENTED_EDGE('',*,*,#6839,.T.);
#9462=ORIENTED_EDGE('',*,*,#6838,.F.);
#9463=ORIENTED_EDGE('',*,*,#6840,.T.);
#9464=ORIENTED_EDGE('',*,*,#6841,.T.);
#9465=ORIENTED_EDGE('',*,*,#6842,.T.);
#9466=ORIENTED_EDGE('',*,*,#6841,.F.);
#9467=ORIENTED_EDGE('',*,*,#6843,.T.);
#9468=ORIENTED_EDGE('',*,*,#6844,.T.);
#9469=ORIENTED_EDGE('',*,*,#6845,.T.);
#9470=ORIENTED_EDGE('',*,*,#6844,.F.);
#10246=CYLINDRICAL_SURFACE('',#11675,1.25);
#10247=CYLINDRICAL_SURFACE('',#11678,1.25);
#10248=CYLINDRICAL_SURFACE('',#11681,1.25);
#10249=CYLINDRICAL_SURFACE('',#11684,1.25);
#10250=CYLINDRICAL_SURFACE('',#11687,1.025);
#10251=CYLINDRICAL_SURFACE('',#11690,1.025);
#10252=CYLINDRICAL_SURFACE('',#11693,1.025);
#10253=CYLINDRICAL_SURFACE('',#11696,1.025);
#10254=CYLINDRICAL_SURFACE('',#11699,1.25);
#10255=CYLINDRICAL_SURFACE('',#11702,1.25);
#10256=CYLINDRICAL_SURFACE('',#11705,1.25);
#10257=CYLINDRICAL_SURFACE('',#11708,1.25);
#10258=CYLINDRICAL_SURFACE('',#11711,1.025);
#10259=CYLINDRICAL_SURFACE('',#11714,1.025);
#10260=CYLINDRICAL_SURFACE('',#11717,1.025);
#10261=CYLINDRICAL_SURFACE('',#11720,1.025);
#10262=CYLINDRICAL_SURFACE('',#11723,1.25);
#10263=CYLINDRICAL_SURFACE('',#11726,1.25);
#10264=CYLINDRICAL_SURFACE('',#11729,1.25);
#10265=CYLINDRICAL_SURFACE('',#11732,1.25);
#10266=CYLINDRICAL_SURFACE('',#11735,1.25);
#10267=CYLINDRICAL_SURFACE('',#11738,1.25);
#10268=CYLINDRICAL_SURFACE('',#11741,1.25);
#10269=CYLINDRICAL_SURFACE('',#11744,1.25);
#10270=CYLINDRICAL_SURFACE('',#11747,5.);
#10271=CYLINDRICAL_SURFACE('',#11768,1.3);
#10272=CYLINDRICAL_SURFACE('',#11771,1.3);
#10273=CYLINDRICAL_SURFACE('',#11774,1.3);
#10274=CYLINDRICAL_SURFACE('',#11777,1.3);
#10275=CYLINDRICAL_SURFACE('',#11780,1.3);
#10276=CYLINDRICAL_SURFACE('',#11783,1.3);
#10277=CYLINDRICAL_SURFACE('',#11786,1.3);
#10278=CYLINDRICAL_SURFACE('',#11789,1.3);
#10279=CYLINDRICAL_SURFACE('',#11795,0.5);
#10280=CYLINDRICAL_SURFACE('',#11802,0.5);
#10281=CYLINDRICAL_SURFACE('',#11804,6.);
#10282=CYLINDRICAL_SURFACE('',#11807,6.);
#10283=CYLINDRICAL_SURFACE('',#11818,2.5);
#10284=CYLINDRICAL_SURFACE('',#11820,2.5);
#10285=CYLINDRICAL_SURFACE('',#11823,2.);
#10286=CYLINDRICAL_SURFACE('',#11825,2.);
#10287=CYLINDRICAL_SURFACE('',#11828,2.);
#10288=CYLINDRICAL_SURFACE('',#11831,2.);
#10289=CYLINDRICAL_SURFACE('',#11833,2.);
#10290=CYLINDRICAL_SURFACE('',#11836,2.);
#10291=CYLINDRICAL_SURFACE('',#11842,1.25);
#10292=CYLINDRICAL_SURFACE('',#11845,1.25);
#10293=CYLINDRICAL_SURFACE('',#11848,1.25);
#10294=CYLINDRICAL_SURFACE('',#11851,1.25);
#10295=CYLINDRICAL_SURFACE('',#11854,1.25);
#10296=CYLINDRICAL_SURFACE('',#11857,1.25);
#10297=CYLINDRICAL_SURFACE('',#11860,1.25);
#10298=CYLINDRICAL_SURFACE('',#11863,1.25);
#10709=ADVANCED_FACE('',(#1257),#10246,.F.);
#10710=ADVANCED_FACE('',(#1258),#10247,.F.);
#10711=ADVANCED_FACE('',(#1259),#10248,.F.);
#10712=ADVANCED_FACE('',(#1260),#10249,.F.);
#10713=ADVANCED_FACE('',(#1261),#10250,.F.);
#10714=ADVANCED_FACE('',(#1262),#10251,.F.);
#10715=ADVANCED_FACE('',(#1263),#10252,.F.);
#10716=ADVANCED_FACE('',(#1264),#10253,.F.);
#10717=ADVANCED_FACE('',(#1265),#10254,.F.);
#10718=ADVANCED_FACE('',(#1266),#10255,.F.);
#10719=ADVANCED_FACE('',(#1267),#10256,.F.);
#10720=ADVANCED_FACE('',(#1268),#10257,.F.);
#10721=ADVANCED_FACE('',(#1269),#10258,.F.);
#10722=ADVANCED_FACE('',(#1270),#10259,.F.);
#10723=ADVANCED_FACE('',(#1271),#10260,.F.);
#10724=ADVANCED_FACE('',(#1272),#10261,.F.);
#10725=ADVANCED_FACE('',(#1273),#10262,.F.);
#10726=ADVANCED_FACE('',(#1274),#10263,.F.);
#10727=ADVANCED_FACE('',(#1275),#10264,.F.);
#10728=ADVANCED_FACE('',(#1276),#10265,.F.);
#10729=ADVANCED_FACE('',(#1277),#10266,.F.);
#10730=ADVANCED_FACE('',(#1278),#10267,.F.);
#10731=ADVANCED_FACE('',(#1279),#10268,.F.);
#10732=ADVANCED_FACE('',(#1280),#10269,.F.);
#10733=ADVANCED_FACE('',(#1281),#10270,.F.);
#10734=ADVANCED_FACE('',(#1282),#205,.F.);
#10735=ADVANCED_FACE('',(#1283),#206,.F.);
#10736=ADVANCED_FACE('',(#1284),#207,.F.);
#10737=ADVANCED_FACE('',(#1285),#208,.F.);
#10738=ADVANCED_FACE('',(#1286),#209,.F.);
#10739=ADVANCED_FACE('',(#1287),#210,.F.);
#10740=ADVANCED_FACE('',(#1288),#211,.F.);
#10741=ADVANCED_FACE('',(#1289),#212,.F.);
#10742=ADVANCED_FACE('',(#1290),#213,.F.);
#10743=ADVANCED_FACE('',(#1291),#10271,.F.);
#10744=ADVANCED_FACE('',(#1292),#10272,.F.);
#10745=ADVANCED_FACE('',(#1293),#10273,.F.);
#10746=ADVANCED_FACE('',(#1294),#10274,.F.);
#10747=ADVANCED_FACE('',(#1295),#10275,.F.);
#10748=ADVANCED_FACE('',(#1296),#10276,.F.);
#10749=ADVANCED_FACE('',(#1297),#10277,.F.);
#10750=ADVANCED_FACE('',(#1298),#10278,.F.);
#10751=ADVANCED_FACE('',(#1299,#450,#451,#452,#453,#454,#455,#456,#457,
#458,#459,#460,#461,#462,#463,#464,#465,#466,#467,#468,#469,#470,#471,#472,
#473,#474),#808,.F.);
#10752=ADVANCED_FACE('',(#1300),#10279,.F.);
#10753=ADVANCED_FACE('',(#1301),#809,.F.);
#10754=ADVANCED_FACE('',(#1302),#10280,.F.);
#10755=ADVANCED_FACE('',(#1303),#10281,.F.);
#10756=ADVANCED_FACE('',(#1304),#810,.T.);
#10757=ADVANCED_FACE('',(#1305),#10282,.F.);
#10758=ADVANCED_FACE('',(#1306,#475,#476,#477,#478,#479,#480,#481,#482,
#483,#484,#485,#486,#487,#488,#489,#490,#491,#492,#493,#494,#495,#496,#497,
#498,#499),#811,.T.);
#10759=ADVANCED_FACE('',(#1307,#500,#501,#502,#503),#812,.F.);
#10760=ADVANCED_FACE('',(#1308),#240,.F.);
#10761=ADVANCED_FACE('',(#1309),#241,.F.);
#10762=ADVANCED_FACE('',(#1310,#504,#505,#506,#507),#813,.F.);
#10763=ADVANCED_FACE('',(#1311),#10283,.T.);
#10764=ADVANCED_FACE('',(#1312),#10284,.T.);
#10765=ADVANCED_FACE('',(#1313),#814,.T.);
#10766=ADVANCED_FACE('',(#1314),#10285,.T.);
#10767=ADVANCED_FACE('',(#1315),#10286,.T.);
#10768=ADVANCED_FACE('',(#1316),#815,.T.);
#10769=ADVANCED_FACE('',(#1317),#10287,.T.);
#10770=ADVANCED_FACE('',(#1318),#242,.F.);
#10771=ADVANCED_FACE('',(#1319),#243,.T.);
#10772=ADVANCED_FACE('',(#1320),#816,.F.);
#10773=ADVANCED_FACE('',(#1321),#10288,.T.);
#10774=ADVANCED_FACE('',(#1322),#10289,.T.);
#10775=ADVANCED_FACE('',(#1323),#817,.T.);
#10776=ADVANCED_FACE('',(#1324),#10290,.T.);
#10777=ADVANCED_FACE('',(#1325,#508,#509,#510,#511),#818,.T.);
#10778=ADVANCED_FACE('',(#1326,#512,#513,#514,#515),#819,.T.);
#10779=ADVANCED_FACE('',(#1327),#820,.T.);
#10780=ADVANCED_FACE('',(#1328),#821,.T.);
#10781=ADVANCED_FACE('',(#1329),#10291,.T.);
#10782=ADVANCED_FACE('',(#1330),#10292,.T.);
#10783=ADVANCED_FACE('',(#1331),#10293,.T.);
#10784=ADVANCED_FACE('',(#1332),#10294,.T.);
#10785=ADVANCED_FACE('',(#1333),#10295,.T.);
#10786=ADVANCED_FACE('',(#1334),#10296,.T.);
#10787=ADVANCED_FACE('',(#1335),#10297,.T.);
#10788=ADVANCED_FACE('',(#1336),#10298,.T.);
#10946=CLOSED_SHELL('',(#10709,#10710,#10711,#10712,#10713,#10714,#10715,
#10716,#10717,#10718,#10719,#10720,#10721,#10722,#10723,#10724,#10725,#10726,
#10727,#10728,#10729,#10730,#10731,#10732,#10733,#10734,#10735,#10736,#10737,
#10738,#10739,#10740,#10741,#10742,#10743,#10744,#10745,#10746,#10747,#10748,
#10749,#10750,#10751,#10752,#10753,#10754,#10755,#10756,#10757,#10758,#10759,
#10760,#10761,#10762,#10763,#10764,#10765,#10766,#10767,#10768,#10769,#10770,
#10771,#10772,#10773,#10774,#10775,#10776,#10777,#10778,#10779,#10780));
#11674=AXIS2_PLACEMENT_3D('',#18751,#14041,#14042);
#11675=AXIS2_PLACEMENT_3D('',#18752,#14043,#14044);
#11676=AXIS2_PLACEMENT_3D('',#18754,#14045,#14046);
#11677=AXIS2_PLACEMENT_3D('',#18757,#14048,#14049);
#11678=AXIS2_PLACEMENT_3D('',#18758,#14050,#14051);
#11679=AXIS2_PLACEMENT_3D('',#18760,#14052,#14053);
#11680=AXIS2_PLACEMENT_3D('',#18763,#14055,#14056);
#11681=AXIS2_PLACEMENT_3D('',#18764,#14057,#14058);
#11682=AXIS2_PLACEMENT_3D('',#18766,#14059,#14060);
#11683=AXIS2_PLACEMENT_3D('',#18769,#14062,#14063);
#11684=AXIS2_PLACEMENT_3D('',#18770,#14064,#14065);
#11685=AXIS2_PLACEMENT_3D('',#18772,#14066,#14067);
#11686=AXIS2_PLACEMENT_3D('',#18775,#14069,#14070);
#11687=AXIS2_PLACEMENT_3D('',#18776,#14071,#14072);
#11688=AXIS2_PLACEMENT_3D('',#18778,#14073,#14074);
#11689=AXIS2_PLACEMENT_3D('',#18781,#14076,#14077);
#11690=AXIS2_PLACEMENT_3D('',#18782,#14078,#14079);
#11691=AXIS2_PLACEMENT_3D('',#18784,#14080,#14081);
#11692=AXIS2_PLACEMENT_3D('',#18787,#14083,#14084);
#11693=AXIS2_PLACEMENT_3D('',#18788,#14085,#14086);
#11694=AXIS2_PLACEMENT_3D('',#18790,#14087,#14088);
#11695=AXIS2_PLACEMENT_3D('',#18793,#14090,#14091);
#11696=AXIS2_PLACEMENT_3D('',#18794,#14092,#14093);
#11697=AXIS2_PLACEMENT_3D('',#18796,#14094,#14095);
#11698=AXIS2_PLACEMENT_3D('',#18799,#14097,#14098);
#11699=AXIS2_PLACEMENT_3D('',#18800,#14099,#14100);
#11700=AXIS2_PLACEMENT_3D('',#18802,#14101,#14102);
#11701=AXIS2_PLACEMENT_3D('',#18805,#14104,#14105);
#11702=AXIS2_PLACEMENT_3D('',#18806,#14106,#14107);
#11703=AXIS2_PLACEMENT_3D('',#18808,#14108,#14109);
#11704=AXIS2_PLACEMENT_3D('',#18811,#14111,#14112);
#11705=AXIS2_PLACEMENT_3D('',#18812,#14113,#14114);
#11706=AXIS2_PLACEMENT_3D('',#18814,#14115,#14116);
#11707=AXIS2_PLACEMENT_3D('',#18817,#14118,#14119);
#11708=AXIS2_PLACEMENT_3D('',#18818,#14120,#14121);
#11709=AXIS2_PLACEMENT_3D('',#18820,#14122,#14123);
#11710=AXIS2_PLACEMENT_3D('',#18823,#14125,#14126);
#11711=AXIS2_PLACEMENT_3D('',#18824,#14127,#14128);
#11712=AXIS2_PLACEMENT_3D('',#18826,#14129,#14130);
#11713=AXIS2_PLACEMENT_3D('',#18829,#14132,#14133);
#11714=AXIS2_PLACEMENT_3D('',#18830,#14134,#14135);
#11715=AXIS2_PLACEMENT_3D('',#18832,#14136,#14137);
#11716=AXIS2_PLACEMENT_3D('',#18835,#14139,#14140);
#11717=AXIS2_PLACEMENT_3D('',#18836,#14141,#14142);
#11718=AXIS2_PLACEMENT_3D('',#18838,#14143,#14144);
#11719=AXIS2_PLACEMENT_3D('',#18841,#14146,#14147);
#11720=AXIS2_PLACEMENT_3D('',#18842,#14148,#14149);
#11721=AXIS2_PLACEMENT_3D('',#18844,#14150,#14151);
#11722=AXIS2_PLACEMENT_3D('',#18847,#14153,#14154);
#11723=AXIS2_PLACEMENT_3D('',#18848,#14155,#14156);
#11724=AXIS2_PLACEMENT_3D('',#18850,#14157,#14158);
#11725=AXIS2_PLACEMENT_3D('',#18853,#14160,#14161);
#11726=AXIS2_PLACEMENT_3D('',#18854,#14162,#14163);
#11727=AXIS2_PLACEMENT_3D('',#18856,#14164,#14165);
#11728=AXIS2_PLACEMENT_3D('',#18859,#14167,#14168);
#11729=AXIS2_PLACEMENT_3D('',#18860,#14169,#14170);
#11730=AXIS2_PLACEMENT_3D('',#18862,#14171,#14172);
#11731=AXIS2_PLACEMENT_3D('',#18865,#14174,#14175);
#11732=AXIS2_PLACEMENT_3D('',#18866,#14176,#14177);
#11733=AXIS2_PLACEMENT_3D('',#18868,#14178,#14179);
#11734=AXIS2_PLACEMENT_3D('',#18871,#14181,#14182);
#11735=AXIS2_PLACEMENT_3D('',#18872,#14183,#14184);
#11736=AXIS2_PLACEMENT_3D('',#18874,#14185,#14186);
#11737=AXIS2_PLACEMENT_3D('',#18877,#14188,#14189);
#11738=AXIS2_PLACEMENT_3D('',#18878,#14190,#14191);
#11739=AXIS2_PLACEMENT_3D('',#18880,#14192,#14193);
#11740=AXIS2_PLACEMENT_3D('',#18883,#14195,#14196);
#11741=AXIS2_PLACEMENT_3D('',#18884,#14197,#14198);
#11742=AXIS2_PLACEMENT_3D('',#18886,#14199,#14200);
#11743=AXIS2_PLACEMENT_3D('',#18889,#14202,#14203);
#11744=AXIS2_PLACEMENT_3D('',#18890,#14204,#14205);
#11745=AXIS2_PLACEMENT_3D('',#18892,#14206,#14207);
#11746=AXIS2_PLACEMENT_3D('',#18895,#14209,#14210);
#11747=AXIS2_PLACEMENT_3D('',#18896,#14211,#14212);
#11748=AXIS2_PLACEMENT_3D('',#18898,#14213,#14214);
#11749=AXIS2_PLACEMENT_3D('',#18901,#14216,#14217);
#11750=AXIS2_PLACEMENT_3D('',#18902,#14218,#14219);
#11751=AXIS2_PLACEMENT_3D('',#18905,#14221,#14222);
#11752=AXIS2_PLACEMENT_3D('',#18906,#14223,#14224);
#11753=AXIS2_PLACEMENT_3D('',#18909,#14226,#14227);
#11754=AXIS2_PLACEMENT_3D('',#18910,#14228,#14229);
#11755=AXIS2_PLACEMENT_3D('',#18913,#14231,#14232);
#11756=AXIS2_PLACEMENT_3D('',#18914,#14233,#14234);
#11757=AXIS2_PLACEMENT_3D('',#18917,#14236,#14237);
#11758=AXIS2_PLACEMENT_3D('',#18918,#14238,#14239);
#11759=AXIS2_PLACEMENT_3D('',#18921,#14241,#14242);
#11760=AXIS2_PLACEMENT_3D('',#18922,#14243,#14244);
#11761=AXIS2_PLACEMENT_3D('',#18925,#14246,#14247);
#11762=AXIS2_PLACEMENT_3D('',#18926,#14248,#14249);
#11763=AXIS2_PLACEMENT_3D('',#18929,#14251,#14252);
#11764=AXIS2_PLACEMENT_3D('',#18930,#14253,#14254);
#11765=AXIS2_PLACEMENT_3D('',#18933,#14256,#14257);
#11766=AXIS2_PLACEMENT_3D('',#18934,#14258,#14259);
#11767=AXIS2_PLACEMENT_3D('',#18937,#14261,#14262);
#11768=AXIS2_PLACEMENT_3D('',#18938,#14263,#14264);
#11769=AXIS2_PLACEMENT_3D('',#18940,#14265,#14266);
#11770=AXIS2_PLACEMENT_3D('',#18943,#14268,#14269);
#11771=AXIS2_PLACEMENT_3D('',#18944,#14270,#14271);
#11772=AXIS2_PLACEMENT_3D('',#18946,#14272,#14273);
#11773=AXIS2_PLACEMENT_3D('',#18949,#14275,#14276);
#11774=AXIS2_PLACEMENT_3D('',#18950,#14277,#14278);
#11775=AXIS2_PLACEMENT_3D('',#18952,#14279,#14280);
#11776=AXIS2_PLACEMENT_3D('',#18955,#14282,#14283);
#11777=AXIS2_PLACEMENT_3D('',#18956,#14284,#14285);
#11778=AXIS2_PLACEMENT_3D('',#18958,#14286,#14287);
#11779=AXIS2_PLACEMENT_3D('',#18961,#14289,#14290);
#11780=AXIS2_PLACEMENT_3D('',#18962,#14291,#14292);
#11781=AXIS2_PLACEMENT_3D('',#18964,#14293,#14294);
#11782=AXIS2_PLACEMENT_3D('',#18967,#14296,#14297);
#11783=AXIS2_PLACEMENT_3D('',#18968,#14298,#14299);
#11784=AXIS2_PLACEMENT_3D('',#18970,#14300,#14301);
#11785=AXIS2_PLACEMENT_3D('',#18973,#14303,#14304);
#11786=AXIS2_PLACEMENT_3D('',#18974,#14305,#14306);
#11787=AXIS2_PLACEMENT_3D('',#18976,#14307,#14308);
#11788=AXIS2_PLACEMENT_3D('',#18979,#14310,#14311);
#11789=AXIS2_PLACEMENT_3D('',#18980,#14312,#14313);
#11790=AXIS2_PLACEMENT_3D('',#18982,#14314,#14315);
#11791=AXIS2_PLACEMENT_3D('',#18985,#14317,#14318);
#11792=AXIS2_PLACEMENT_3D('',#18986,#14319,#14320);
#11793=AXIS2_PLACEMENT_3D('',#18993,#14323,#14324);
#11794=AXIS2_PLACEMENT_3D('',#18997,#14326,#14327);
#11795=AXIS2_PLACEMENT_3D('',#18999,#14329,#14330);
#11796=AXIS2_PLACEMENT_3D('',#19001,#14331,#14332);
#11797=AXIS2_PLACEMENT_3D('',#19018,#14333,#14334);
#11798=AXIS2_PLACEMENT_3D('',#19020,#14336,#14337);
#11799=AXIS2_PLACEMENT_3D('',#19028,#14341,#14342);
#11800=AXIS2_PLACEMENT_3D('',#19032,#14344,#14345);
#11801=AXIS2_PLACEMENT_3D('',#19039,#14349,#14350);
#11802=AXIS2_PLACEMENT_3D('',#19040,#14351,#14352);
#11803=AXIS2_PLACEMENT_3D('',#19044,#14354,#14355);
#11804=AXIS2_PLACEMENT_3D('',#19059,#14356,#14357);
#11805=AXIS2_PLACEMENT_3D('',#19065,#14360,#14361);
#11806=AXIS2_PLACEMENT_3D('',#19067,#14363,#14364);
#11807=AXIS2_PLACEMENT_3D('',#19071,#14367,#14368);
#11808=AXIS2_PLACEMENT_3D('',#19073,#14369,#14370);
#11809=AXIS2_PLACEMENT_3D('',#19077,#14373,#14374);
#11810=AXIS2_PLACEMENT_3D('',#19080,#14377,#14378);
#11811=AXIS2_PLACEMENT_3D('',#19084,#14380,#14381);
#11812=AXIS2_PLACEMENT_3D('',#19088,#14383,#14384);
#11813=AXIS2_PLACEMENT_3D('',#19091,#14386,#14387);
#11814=AXIS2_PLACEMENT_3D('',#19196,#14390,#14391);
#11815=AXIS2_PLACEMENT_3D('',#19199,#14392,#14393);
#11816=AXIS2_PLACEMENT_3D('',#19203,#14395,#14396);
#11817=AXIS2_PLACEMENT_3D('',#19206,#14398,#14399);
#11818=AXIS2_PLACEMENT_3D('',#19208,#14401,#14402);
#11819=AXIS2_PLACEMENT_3D('',#19211,#14404,#14405);
#11820=AXIS2_PLACEMENT_3D('',#19212,#14406,#14407);
#11821=AXIS2_PLACEMENT_3D('',#19214,#14408,#14409);
#11822=AXIS2_PLACEMENT_3D('',#19216,#14411,#14412);
#11823=AXIS2_PLACEMENT_3D('',#19223,#14417,#14418);
#11824=AXIS2_PLACEMENT_3D('',#19225,#14419,#14420);
#11825=AXIS2_PLACEMENT_3D('',#19227,#14422,#14423);
#11826=AXIS2_PLACEMENT_3D('',#19231,#14425,#14426);
#11827=AXIS2_PLACEMENT_3D('',#19233,#14428,#14429);
#11828=AXIS2_PLACEMENT_3D('',#19237,#14432,#14433);
#11829=AXIS2_PLACEMENT_3D('',#19238,#14434,#14435);
#11830=AXIS2_PLACEMENT_3D('',#19290,#14438,#14439);
#11831=AXIS2_PLACEMENT_3D('',#19296,#14443,#14444);
#11832=AXIS2_PLACEMENT_3D('',#19298,#14445,#14446);
#11833=AXIS2_PLACEMENT_3D('',#19300,#14448,#14449);
#11834=AXIS2_PLACEMENT_3D('',#19304,#14451,#14452);
#11835=AXIS2_PLACEMENT_3D('',#19306,#14454,#14455);
#11836=AXIS2_PLACEMENT_3D('',#19308,#14457,#14458);
#11837=AXIS2_PLACEMENT_3D('',#19309,#14459,#14460);
#11838=AXIS2_PLACEMENT_3D('',#19310,#14461,#14462);
#11839=AXIS2_PLACEMENT_3D('',#19312,#14464,#14465);
#11840=AXIS2_PLACEMENT_3D('',#19314,#14467,#14468);
#11841=AXIS2_PLACEMENT_3D('',#19315,#14469,#14470);
#11842=AXIS2_PLACEMENT_3D('',#19316,#14471,#14472);
#11843=AXIS2_PLACEMENT_3D('',#19318,#14473,#14474);
#11844=AXIS2_PLACEMENT_3D('',#19321,#14476,#14477);
#11845=AXIS2_PLACEMENT_3D('',#19322,#14478,#14479);
#11846=AXIS2_PLACEMENT_3D('',#19324,#14480,#14481);
#11847=AXIS2_PLACEMENT_3D('',#19327,#14483,#14484);
#11848=AXIS2_PLACEMENT_3D('',#19328,#14485,#14486);
#11849=AXIS2_PLACEMENT_3D('',#19330,#14487,#14488);
#11850=AXIS2_PLACEMENT_3D('',#19333,#14490,#14491);
#11851=AXIS2_PLACEMENT_3D('',#19334,#14492,#14493);
#11852=AXIS2_PLACEMENT_3D('',#19336,#14494,#14495);
#11853=AXIS2_PLACEMENT_3D('',#19339,#14497,#14498);
#11854=AXIS2_PLACEMENT_3D('',#19340,#14499,#14500);
#11855=AXIS2_PLACEMENT_3D('',#19342,#14501,#14502);
#11856=AXIS2_PLACEMENT_3D('',#19345,#14504,#14505);
#11857=AXIS2_PLACEMENT_3D('',#19346,#14506,#14507);
#11858=AXIS2_PLACEMENT_3D('',#19348,#14508,#14509);
#11859=AXIS2_PLACEMENT_3D('',#19351,#14511,#14512);
#11860=AXIS2_PLACEMENT_3D('',#19352,#14513,#14514);
#11861=AXIS2_PLACEMENT_3D('',#19354,#14515,#14516);
#11862=AXIS2_PLACEMENT_3D('',#19357,#14518,#14519);
#11863=AXIS2_PLACEMENT_3D('',#19358,#14520,#14521);
#11864=AXIS2_PLACEMENT_3D('',#19360,#14522,#14523);
#11865=AXIS2_PLACEMENT_3D('',#19363,#14525,#14526);
#14041=DIRECTION('axis',(0.,0.,1.));
#14042=DIRECTION('refdir',(1.,0.,0.));
#14043=DIRECTION('center_axis',(0.,1.,0.));
#14044=DIRECTION('ref_axis',(0.,0.,1.));
#14045=DIRECTION('center_axis',(0.,1.,0.));
#14046=DIRECTION('ref_axis',(0.,0.,1.));
#14047=DIRECTION('',(0.,1.,0.));
#14048=DIRECTION('center_axis',(0.,1.,0.));
#14049=DIRECTION('ref_axis',(0.,0.,1.));
#14050=DIRECTION('center_axis',(0.,1.,0.));
#14051=DIRECTION('ref_axis',(0.,0.,1.));
#14052=DIRECTION('center_axis',(0.,1.,0.));
#14053=DIRECTION('ref_axis',(0.,0.,1.));
#14054=DIRECTION('',(0.,1.,0.));
#14055=DIRECTION('center_axis',(0.,1.,0.));
#14056=DIRECTION('ref_axis',(0.,0.,1.));
#14057=DIRECTION('center_axis',(0.,1.,0.));
#14058=DIRECTION('ref_axis',(0.,0.,1.));
#14059=DIRECTION('center_axis',(0.,1.,0.));
#14060=DIRECTION('ref_axis',(0.,0.,1.));
#14061=DIRECTION('',(0.,1.,0.));
#14062=DIRECTION('center_axis',(0.,1.,0.));
#14063=DIRECTION('ref_axis',(0.,0.,1.));
#14064=DIRECTION('center_axis',(0.,1.,0.));
#14065=DIRECTION('ref_axis',(0.,0.,1.));
#14066=DIRECTION('center_axis',(0.,1.,0.));
#14067=DIRECTION('ref_axis',(0.,0.,1.));
#14068=DIRECTION('',(0.,1.,0.));
#14069=DIRECTION('center_axis',(0.,1.,0.));
#14070=DIRECTION('ref_axis',(0.,0.,1.));
#14071=DIRECTION('center_axis',(0.,-1.,0.));
#14072=DIRECTION('ref_axis',(0.,0.,-1.));
#14073=DIRECTION('center_axis',(0.,1.,0.));
#14074=DIRECTION('ref_axis',(0.,0.,-1.));
#14075=DIRECTION('',(0.,-1.,0.));
#14076=DIRECTION('center_axis',(0.,1.,0.));
#14077=DIRECTION('ref_axis',(0.,0.,-1.));
#14078=DIRECTION('center_axis',(0.,-1.,0.));
#14079=DIRECTION('ref_axis',(0.,0.,-1.));
#14080=DIRECTION('center_axis',(0.,1.,0.));
#14081=DIRECTION('ref_axis',(0.,0.,-1.));
#14082=DIRECTION('',(0.,-1.,0.));
#14083=DIRECTION('center_axis',(0.,1.,0.));
#14084=DIRECTION('ref_axis',(0.,0.,-1.));
#14085=DIRECTION('center_axis',(0.,-1.,0.));
#14086=DIRECTION('ref_axis',(0.,0.,-1.));
#14087=DIRECTION('center_axis',(0.,1.,0.));
#14088=DIRECTION('ref_axis',(0.,0.,-1.));
#14089=DIRECTION('',(0.,-1.,0.));
#14090=DIRECTION('center_axis',(0.,1.,0.));
#14091=DIRECTION('ref_axis',(0.,0.,-1.));
#14092=DIRECTION('center_axis',(0.,-1.,0.));
#14093=DIRECTION('ref_axis',(0.,0.,-1.));
#14094=DIRECTION('center_axis',(0.,1.,0.));
#14095=DIRECTION('ref_axis',(0.,0.,-1.));
#14096=DIRECTION('',(0.,-1.,0.));
#14097=DIRECTION('center_axis',(0.,1.,0.));
#14098=DIRECTION('ref_axis',(0.,0.,-1.));
#14099=DIRECTION('center_axis',(0.,1.,0.));
#14100=DIRECTION('ref_axis',(0.,0.,1.));
#14101=DIRECTION('center_axis',(0.,1.,0.));
#14102=DIRECTION('ref_axis',(0.,0.,1.));
#14103=DIRECTION('',(0.,1.,0.));
#14104=DIRECTION('center_axis',(0.,1.,0.));
#14105=DIRECTION('ref_axis',(0.,0.,1.));
#14106=DIRECTION('center_axis',(0.,1.,0.));
#14107=DIRECTION('ref_axis',(0.,0.,1.));
#14108=DIRECTION('center_axis',(0.,1.,0.));
#14109=DIRECTION('ref_axis',(0.,0.,1.));
#14110=DIRECTION('',(0.,1.,0.));
#14111=DIRECTION('center_axis',(0.,1.,0.));
#14112=DIRECTION('ref_axis',(0.,0.,1.));
#14113=DIRECTION('center_axis',(0.,1.,0.));
#14114=DIRECTION('ref_axis',(0.,0.,1.));
#14115=DIRECTION('center_axis',(0.,1.,0.));
#14116=DIRECTION('ref_axis',(0.,0.,1.));
#14117=DIRECTION('',(0.,1.,0.));
#14118=DIRECTION('center_axis',(0.,1.,0.));
#14119=DIRECTION('ref_axis',(0.,0.,1.));
#14120=DIRECTION('center_axis',(0.,1.,0.));
#14121=DIRECTION('ref_axis',(0.,0.,1.));
#14122=DIRECTION('center_axis',(0.,1.,0.));
#14123=DIRECTION('ref_axis',(0.,0.,1.));
#14124=DIRECTION('',(0.,1.,0.));
#14125=DIRECTION('center_axis',(0.,1.,0.));
#14126=DIRECTION('ref_axis',(0.,0.,1.));
#14127=DIRECTION('center_axis',(0.,-1.,0.));
#14128=DIRECTION('ref_axis',(0.,0.,-1.));
#14129=DIRECTION('center_axis',(0.,1.,0.));
#14130=DIRECTION('ref_axis',(0.,0.,-1.));
#14131=DIRECTION('',(0.,-1.,0.));
#14132=DIRECTION('center_axis',(0.,1.,0.));
#14133=DIRECTION('ref_axis',(0.,0.,-1.));
#14134=DIRECTION('center_axis',(0.,-1.,0.));
#14135=DIRECTION('ref_axis',(0.,0.,-1.));
#14136=DIRECTION('center_axis',(0.,1.,0.));
#14137=DIRECTION('ref_axis',(0.,0.,-1.));
#14138=DIRECTION('',(0.,-1.,0.));
#14139=DIRECTION('center_axis',(0.,1.,0.));
#14140=DIRECTION('ref_axis',(0.,0.,-1.));
#14141=DIRECTION('center_axis',(0.,-1.,0.));
#14142=DIRECTION('ref_axis',(0.,0.,-1.));
#14143=DIRECTION('center_axis',(0.,1.,0.));
#14144=DIRECTION('ref_axis',(0.,0.,-1.));
#14145=DIRECTION('',(0.,-1.,0.));
#14146=DIRECTION('center_axis',(0.,1.,0.));
#14147=DIRECTION('ref_axis',(0.,0.,-1.));
#14148=DIRECTION('center_axis',(0.,-1.,0.));
#14149=DIRECTION('ref_axis',(0.,0.,-1.));
#14150=DIRECTION('center_axis',(0.,1.,0.));
#14151=DIRECTION('ref_axis',(0.,0.,-1.));
#14152=DIRECTION('',(0.,-1.,0.));
#14153=DIRECTION('center_axis',(0.,1.,0.));
#14154=DIRECTION('ref_axis',(0.,0.,-1.));
#14155=DIRECTION('center_axis',(0.,-1.,0.));
#14156=DIRECTION('ref_axis',(0.,0.,-1.));
#14157=DIRECTION('center_axis',(0.,1.,0.));
#14158=DIRECTION('ref_axis',(0.,0.,-1.));
#14159=DIRECTION('',(0.,-1.,0.));
#14160=DIRECTION('center_axis',(0.,1.,0.));
#14161=DIRECTION('ref_axis',(0.,0.,-1.));
#14162=DIRECTION('center_axis',(0.,-1.,0.));
#14163=DIRECTION('ref_axis',(0.,0.,-1.));
#14164=DIRECTION('center_axis',(0.,1.,0.));
#14165=DIRECTION('ref_axis',(0.,0.,-1.));
#14166=DIRECTION('',(0.,-1.,0.));
#14167=DIRECTION('center_axis',(0.,1.,0.));
#14168=DIRECTION('ref_axis',(0.,0.,-1.));
#14169=DIRECTION('center_axis',(0.,-1.,0.));
#14170=DIRECTION('ref_axis',(0.,0.,-1.));
#14171=DIRECTION('center_axis',(0.,1.,0.));
#14172=DIRECTION('ref_axis',(0.,0.,-1.));
#14173=DIRECTION('',(0.,-1.,0.));
#14174=DIRECTION('center_axis',(0.,1.,0.));
#14175=DIRECTION('ref_axis',(0.,0.,-1.));
#14176=DIRECTION('center_axis',(0.,-1.,0.));
#14177=DIRECTION('ref_axis',(0.,0.,-1.));
#14178=DIRECTION('center_axis',(0.,1.,0.));
#14179=DIRECTION('ref_axis',(0.,0.,-1.));
#14180=DIRECTION('',(0.,-1.,0.));
#14181=DIRECTION('center_axis',(0.,1.,0.));
#14182=DIRECTION('ref_axis',(0.,0.,-1.));
#14183=DIRECTION('center_axis',(0.,-1.,0.));
#14184=DIRECTION('ref_axis',(0.,0.,-1.));
#14185=DIRECTION('center_axis',(0.,1.,0.));
#14186=DIRECTION('ref_axis',(0.,0.,-1.));
#14187=DIRECTION('',(0.,-1.,0.));
#14188=DIRECTION('center_axis',(0.,1.,0.));
#14189=DIRECTION('ref_axis',(0.,0.,-1.));
#14190=DIRECTION('center_axis',(0.,-1.,0.));
#14191=DIRECTION('ref_axis',(0.,0.,-1.));
#14192=DIRECTION('center_axis',(0.,1.,0.));
#14193=DIRECTION('ref_axis',(0.,0.,-1.));
#14194=DIRECTION('',(0.,-1.,0.));
#14195=DIRECTION('center_axis',(0.,1.,0.));
#14196=DIRECTION('ref_axis',(0.,0.,-1.));
#14197=DIRECTION('center_axis',(0.,-1.,0.));
#14198=DIRECTION('ref_axis',(0.,0.,-1.));
#14199=DIRECTION('center_axis',(0.,1.,0.));
#14200=DIRECTION('ref_axis',(0.,0.,-1.));
#14201=DIRECTION('',(0.,-1.,0.));
#14202=DIRECTION('center_axis',(0.,1.,0.));
#14203=DIRECTION('ref_axis',(0.,0.,-1.));
#14204=DIRECTION('center_axis',(0.,-1.,0.));
#14205=DIRECTION('ref_axis',(0.,0.,-1.));
#14206=DIRECTION('center_axis',(0.,1.,0.));
#14207=DIRECTION('ref_axis',(0.,0.,-1.));
#14208=DIRECTION('',(0.,-1.,0.));
#14209=DIRECTION('center_axis',(0.,1.,0.));
#14210=DIRECTION('ref_axis',(0.,0.,-1.));
#14211=DIRECTION('center_axis',(0.,-1.,0.));
#14212=DIRECTION('ref_axis',(0.,0.,-1.));
#14213=DIRECTION('center_axis',(0.,1.,0.));
#14214=DIRECTION('ref_axis',(0.,0.,-1.));
#14215=DIRECTION('',(0.,-1.,0.));
#14216=DIRECTION('center_axis',(0.,1.,0.));
#14217=DIRECTION('ref_axis',(0.,0.,-1.));
#14218=DIRECTION('center_axis',(0.,-1.,0.));
#14219=DIRECTION('ref_axis',(0.,0.,-1.));
#14220=DIRECTION('',(-8.65956056235493E-17,-0.707106781186548,0.707106781186547));
#14221=DIRECTION('center_axis',(0.,1.,0.));
#14222=DIRECTION('ref_axis',(0.,0.,-1.));
#14223=DIRECTION('center_axis',(0.,-1.,0.));
#14224=DIRECTION('ref_axis',(0.,0.,-1.));
#14225=DIRECTION('',(-8.65956056235493E-17,-0.707106781186548,0.707106781186547));
#14226=DIRECTION('center_axis',(0.,1.,0.));
#14227=DIRECTION('ref_axis',(0.,0.,-1.));
#14228=DIRECTION('center_axis',(0.,-1.,0.));
#14229=DIRECTION('ref_axis',(0.,0.,-1.));
#14230=DIRECTION('',(-8.65956056235493E-17,-0.707106781186548,0.707106781186547));
#14231=DIRECTION('center_axis',(0.,1.,0.));
#14232=DIRECTION('ref_axis',(0.,0.,-1.));
#14233=DIRECTION('center_axis',(0.,-1.,0.));
#14234=DIRECTION('ref_axis',(0.,0.,-1.));
#14235=DIRECTION('',(-8.65956056235493E-17,-0.707106781186548,0.707106781186547));
#14236=DIRECTION('center_axis',(0.,1.,0.));
#14237=DIRECTION('ref_axis',(0.,0.,-1.));
#14238=DIRECTION('center_axis',(0.,-1.,0.));
#14239=DIRECTION('ref_axis',(0.,0.,-1.));
#14240=DIRECTION('',(-8.65956056235493E-17,-0.707106781186547,0.707106781186547));
#14241=DIRECTION('center_axis',(0.,1.,0.));
#14242=DIRECTION('ref_axis',(0.,0.,-1.));
#14243=DIRECTION('center_axis',(0.,-1.,0.));
#14244=DIRECTION('ref_axis',(0.,0.,-1.));
#14245=DIRECTION('',(-8.65956056235493E-17,-0.707106781186547,0.707106781186547));
#14246=DIRECTION('center_axis',(0.,1.,0.));
#14247=DIRECTION('ref_axis',(0.,0.,-1.));
#14248=DIRECTION('center_axis',(0.,-1.,0.));
#14249=DIRECTION('ref_axis',(0.,0.,-1.));
#14250=DIRECTION('',(-8.65956056235493E-17,-0.707106781186547,0.707106781186547));
#14251=DIRECTION('center_axis',(0.,1.,0.));
#14252=DIRECTION('ref_axis',(0.,0.,-1.));
#14253=DIRECTION('center_axis',(0.,-1.,0.));
#14254=DIRECTION('ref_axis',(0.,0.,-1.));
#14255=DIRECTION('',(-8.65956056235493E-17,-0.707106781186548,0.707106781186547));
#14256=DIRECTION('center_axis',(0.,1.,0.));
#14257=DIRECTION('ref_axis',(0.,0.,-1.));
#14258=DIRECTION('center_axis',(0.,-1.,0.));
#14259=DIRECTION('ref_axis',(0.,0.,-1.));
#14260=DIRECTION('',(-8.65951884466615E-17,-0.707110187677941,0.707103374678744));
#14261=DIRECTION('center_axis',(0.,1.,0.));
#14262=DIRECTION('ref_axis',(0.,0.,-1.));
#14263=DIRECTION('center_axis',(0.,0.,-1.));
#14264=DIRECTION('ref_axis',(-1.,0.,0.));
#14265=DIRECTION('center_axis',(0.,0.,-1.));
#14266=DIRECTION('ref_axis',(-1.,0.,0.));
#14267=DIRECTION('',(0.,0.,-1.));
#14268=DIRECTION('center_axis',(0.,0.,-1.));
#14269=DIRECTION('ref_axis',(-1.,0.,0.));
#14270=DIRECTION('center_axis',(0.,0.,-1.));
#14271=DIRECTION('ref_axis',(-1.,0.,0.));
#14272=DIRECTION('center_axis',(0.,0.,-1.));
#14273=DIRECTION('ref_axis',(-1.,0.,0.));
#14274=DIRECTION('',(0.,0.,-1.));
#14275=DIRECTION('center_axis',(0.,0.,-1.));
#14276=DIRECTION('ref_axis',(-1.,0.,0.));
#14277=DIRECTION('center_axis',(0.,0.,-1.));
#14278=DIRECTION('ref_axis',(-1.,0.,0.));
#14279=DIRECTION('center_axis',(0.,0.,-1.));
#14280=DIRECTION('ref_axis',(-1.,0.,0.));
#14281=DIRECTION('',(0.,0.,-1.));
#14282=DIRECTION('center_axis',(0.,0.,-1.));
#14283=DIRECTION('ref_axis',(-1.,0.,0.));
#14284=DIRECTION('center_axis',(0.,0.,-1.));
#14285=DIRECTION('ref_axis',(-1.,0.,0.));
#14286=DIRECTION('center_axis',(0.,0.,-1.));
#14287=DIRECTION('ref_axis',(-1.,0.,0.));
#14288=DIRECTION('',(0.,0.,-1.));
#14289=DIRECTION('center_axis',(0.,0.,-1.));
#14290=DIRECTION('ref_axis',(-1.,0.,0.));
#14291=DIRECTION('center_axis',(0.,0.,-1.));
#14292=DIRECTION('ref_axis',(-1.,0.,0.));
#14293=DIRECTION('center_axis',(0.,0.,1.));
#14294=DIRECTION('ref_axis',(-1.,0.,0.));
#14295=DIRECTION('',(0.,0.,-1.));
#14296=DIRECTION('center_axis',(0.,0.,1.));
#14297=DIRECTION('ref_axis',(-1.,0.,0.));
#14298=DIRECTION('center_axis',(0.,0.,-1.));
#14299=DIRECTION('ref_axis',(-1.,0.,0.));
#14300=DIRECTION('center_axis',(0.,0.,1.));
#14301=DIRECTION('ref_axis',(-1.,0.,0.));
#14302=DIRECTION('',(0.,0.,-1.));
#14303=DIRECTION('center_axis',(0.,0.,1.));
#14304=DIRECTION('ref_axis',(-1.,0.,0.));
#14305=DIRECTION('center_axis',(0.,0.,-1.));
#14306=DIRECTION('ref_axis',(-1.,0.,0.));
#14307=DIRECTION('center_axis',(0.,0.,1.));
#14308=DIRECTION('ref_axis',(-1.,0.,0.));
#14309=DIRECTION('',(0.,0.,-1.));
#14310=DIRECTION('center_axis',(0.,0.,1.));
#14311=DIRECTION('ref_axis',(-1.,0.,0.));
#14312=DIRECTION('center_axis',(0.,0.,-1.));
#14313=DIRECTION('ref_axis',(-1.,0.,0.));
#14314=DIRECTION('center_axis',(0.,0.,1.));
#14315=DIRECTION('ref_axis',(-1.,0.,0.));
#14316=DIRECTION('',(0.,0.,-1.));
#14317=DIRECTION('center_axis',(0.,0.,1.));
#14318=DIRECTION('ref_axis',(-1.,0.,0.));
#14319=DIRECTION('center_axis',(0.,-1.,0.));
#14320=DIRECTION('ref_axis',(0.,0.,-1.));
#14321=DIRECTION('',(0.,0.,1.));
#14322=DIRECTION('',(1.,0.,0.));
#14323=DIRECTION('center_axis',(0.,1.,0.));
#14324=DIRECTION('ref_axis',(1.73472347597681E-15,0.,-1.));
#14325=DIRECTION('',(0.,0.,-1.));
#14326=DIRECTION('center_axis',(0.,1.,0.));
#14327=DIRECTION('ref_axis',(0.,0.,-1.));
#14328=DIRECTION('',(-1.,0.,0.));
#14329=DIRECTION('center_axis',(1.,0.,0.));
#14330=DIRECTION('ref_axis',(0.,0.,-1.));
#14331=DIRECTION('center_axis',(1.,0.,0.));
#14332=DIRECTION('ref_axis',(0.,0.,-1.));
#14333=DIRECTION('center_axis',(-0.246140467955622,-0.968967287951173,-0.0227434587329154));
#14334=DIRECTION('ref_axis',(0.96923416677013,-0.246072692904075,-0.00577579192399951));
#14335=DIRECTION('',(-1.,0.,0.));
#14336=DIRECTION('center_axis',(-1.,0.,0.));
#14337=DIRECTION('ref_axis',(0.,0.,1.));
#14338=DIRECTION('',(0.,1.,0.));
#14339=DIRECTION('',(0.,0.,-1.));
#14340=DIRECTION('',(0.,1.,0.));
#14341=DIRECTION('center_axis',(-1.,0.,0.));
#14342=DIRECTION('ref_axis',(0.,0.,-1.));
#14343=DIRECTION('',(0.,0.,1.));
#14344=DIRECTION('center_axis',(-1.,0.,0.));
#14345=DIRECTION('ref_axis',(0.,0.,-1.));
#14346=DIRECTION('',(0.,-1.,0.));
#14347=DIRECTION('',(0.,0.,-1.));
#14348=DIRECTION('',(0.,-1.,0.));
#14349=DIRECTION('center_axis',(-1.,0.,0.));
#14350=DIRECTION('ref_axis',(0.,0.,-1.));
#14351=DIRECTION('center_axis',(1.,0.,0.));
#14352=DIRECTION('ref_axis',(0.,0.,-1.));
#14353=DIRECTION('',(1.,0.,0.));
#14354=DIRECTION('center_axis',(0.246140467946646,0.968967287891977,-0.0227434613520755));
#14355=DIRECTION('ref_axis',(0.969234166772409,-0.246072692990846,0.0057757878446833));
#14356=DIRECTION('center_axis',(0.,-1.,0.));
#14357=DIRECTION('ref_axis',(0.,0.,-1.));
#14358=DIRECTION('',(0.,1.,0.));
#14359=DIRECTION('',(0.,1.,0.));
#14360=DIRECTION('center_axis',(0.,1.,0.));
#14361=DIRECTION('ref_axis',(-1.15648231731787E-15,0.,-1.));
#14362=DIRECTION('',(0.,-1.,0.));
#14363=DIRECTION('center_axis',(-1.,0.,0.));
#14364=DIRECTION('ref_axis',(0.,0.,1.));
#14365=DIRECTION('',(0.,0.,1.));
#14366=DIRECTION('',(0.,1.,0.));
#14367=DIRECTION('center_axis',(0.,-1.,0.));
#14368=DIRECTION('ref_axis',(0.,0.,-1.));
#14369=DIRECTION('center_axis',(0.,1.,0.));
#14370=DIRECTION('ref_axis',(0.,0.,-1.));
#14371=DIRECTION('',(0.,-1.,0.));
#14372=DIRECTION('',(0.,-1.,0.));
#14373=DIRECTION('center_axis',(0.,-1.,0.));
#14374=DIRECTION('ref_axis',(0.,0.,-1.));
#14375=DIRECTION('',(-1.,0.,0.));
#14376=DIRECTION('',(1.,0.,0.));
#14377=DIRECTION('center_axis',(0.,0.,1.));
#14378=DIRECTION('ref_axis',(1.,0.,0.));
#14379=DIRECTION('',(0.866025403784817,-0.499999999999345,0.));
#14380=DIRECTION('center_axis',(0.,0.,1.));
#14381=DIRECTION('ref_axis',(1.,0.,0.));
#14382=DIRECTION('',(0.,-1.,0.));
#14383=DIRECTION('center_axis',(0.,0.,1.));
#14384=DIRECTION('ref_axis',(1.,0.,0.));
#14385=DIRECTION('',(-1.,0.,0.));
#14386=DIRECTION('center_axis',(0.,0.,1.));
#14387=DIRECTION('ref_axis',(1.,0.,0.));
#14388=DIRECTION('',(0.,-0.0469178636304674,0.998898750661123));
#14389=DIRECTION('',(0.,0.046917863628385,0.998898750661221));
#14390=DIRECTION('center_axis',(0.,0.,-1.));
#14391=DIRECTION('ref_axis',(-1.,0.,0.));
#14392=DIRECTION('center_axis',(0.,0.,-1.));
#14393=DIRECTION('ref_axis',(-1.,0.,0.));
#14394=DIRECTION('',(0.,1.,0.));
#14395=DIRECTION('center_axis',(0.,0.,-1.));
#14396=DIRECTION('ref_axis',(-1.,0.,0.));
#14397=DIRECTION('',(-0.866025403784817,0.499999999999345,0.));
#14398=DIRECTION('center_axis',(0.,0.,-1.));
#14399=DIRECTION('ref_axis',(-1.,0.,0.));
#14400=DIRECTION('',(1.,0.,0.));
#14401=DIRECTION('center_axis',(1.,0.,0.));
#14402=DIRECTION('ref_axis',(0.,0.,-1.));
#14403=DIRECTION('',(-1.,0.,0.));
#14404=DIRECTION('center_axis',(0.785618915719221,0.618540328946539,0.0145182895295127));
#14405=DIRECTION('ref_axis',(0.0114064440257488,-0.0379409523114369,0.999214880379785));
#14406=DIRECTION('center_axis',(1.,0.,0.));
#14407=DIRECTION('ref_axis',(0.,0.,-1.));
#14408=DIRECTION('center_axis',(0.785618915707418,0.618540328961463,-0.0145182895323779));
#14409=DIRECTION('ref_axis',(-0.0114064440275411,-0.00898185763283676,-0.999894604079905));
#14410=DIRECTION('',(1.,0.,0.));
#14411=DIRECTION('center_axis',(-0.500000000000017,-0.866025403784429,0.));
#14412=DIRECTION('ref_axis',(0.866025403784429,-0.500000000000017,0.));
#14413=DIRECTION('',(-0.866025403784429,0.500000000000017,0.));
#14414=DIRECTION('',(0.,0.,-1.));
#14415=DIRECTION('',(0.,0.,1.));
#14416=DIRECTION('',(0.,0.,1.));
#14417=DIRECTION('center_axis',(0.,0.,1.));
#14418=DIRECTION('ref_axis',(1.,0.,0.));
#14419=DIRECTION('center_axis',(0.,0.,-1.));
#14420=DIRECTION('ref_axis',(1.,1.73472347597681E-15,0.));
#14421=DIRECTION('',(0.,0.,-1.));
#14422=DIRECTION('center_axis',(0.,0.,1.));
#14423=DIRECTION('ref_axis',(1.,0.,0.));
#14424=DIRECTION('',(0.,0.,1.));
#14425=DIRECTION('center_axis',(0.,0.,-1.));
#14426=DIRECTION('ref_axis',(1.,0.,0.));
#14427=DIRECTION('',(0.,0.,-1.));
#14428=DIRECTION('center_axis',(0.,1.,0.));
#14429=DIRECTION('ref_axis',(0.,0.,1.));
#14430=DIRECTION('',(1.,0.,0.));
#14431=DIRECTION('',(0.,0.,-1.));
#14432=DIRECTION('center_axis',(0.,0.,1.));
#14433=DIRECTION('ref_axis',(1.,0.,0.));
#14434=DIRECTION('center_axis',(0.,0.,-1.));
#14435=DIRECTION('ref_axis',(1.,0.,0.));
#14436=DIRECTION('',(0.,-1.85865077509542E-12,-1.));
#14437=DIRECTION('',(0.,-1.85865077509542E-12,-1.));
#14438=DIRECTION('center_axis',(0.,-1.,0.));
#14439=DIRECTION('ref_axis',(0.,0.,-1.));
#14440=DIRECTION('',(0.,0.,-1.));
#14441=DIRECTION('',(0.,0.,1.));
#14442=DIRECTION('',(1.,0.,0.));
#14443=DIRECTION('center_axis',(0.,0.,-1.));
#14444=DIRECTION('ref_axis',(-1.,0.,0.));
#14445=DIRECTION('center_axis',(0.,0.,1.));
#14446=DIRECTION('ref_axis',(-1.,0.,0.));
#14447=DIRECTION('',(0.,0.,1.));
#14448=DIRECTION('center_axis',(0.,0.,-1.));
#14449=DIRECTION('ref_axis',(-1.,0.,0.));
#14450=DIRECTION('',(0.,0.,-1.));
#14451=DIRECTION('center_axis',(0.,0.,1.));
#14452=DIRECTION('ref_axis',(-1.,0.,0.));
#14453=DIRECTION('',(0.,0.,1.));
#14454=DIRECTION('center_axis',(-0.500000000000017,-0.866025403784429,0.));
#14455=DIRECTION('ref_axis',(0.866025403784429,-0.500000000000017,0.));
#14456=DIRECTION('',(0.866025403784429,-0.500000000000017,0.));
#14457=DIRECTION('center_axis',(0.,0.,-1.));
#14458=DIRECTION('ref_axis',(-1.,0.,0.));
#14459=DIRECTION('center_axis',(0.,0.,1.));
#14460=DIRECTION('ref_axis',(-1.,0.,0.));
#14461=DIRECTION('center_axis',(0.,0.,1.));
#14462=DIRECTION('ref_axis',(1.,0.,0.));
#14463=DIRECTION('',(0.,-1.,0.));
#14464=DIRECTION('center_axis',(0.,0.,-1.));
#14465=DIRECTION('ref_axis',(-1.,0.,0.));
#14466=DIRECTION('',(0.,1.,0.));
#14467=DIRECTION('center_axis',(-1.,0.,0.));
#14468=DIRECTION('ref_axis',(0.,0.,1.));
#14469=DIRECTION('center_axis',(-1.,0.,0.));
#14470=DIRECTION('ref_axis',(0.,0.,1.));
#14471=DIRECTION('center_axis',(0.,-1.,0.));
#14472=DIRECTION('ref_axis',(0.,0.,-1.));
#14473=DIRECTION('center_axis',(0.,1.,0.));
#14474=DIRECTION('ref_axis',(0.,0.,-1.));
#14475=DIRECTION('',(0.,1.,0.));
#14476=DIRECTION('center_axis',(0.,-1.,0.));
#14477=DIRECTION('ref_axis',(0.,0.,-1.));
#14478=DIRECTION('center_axis',(0.,-1.,0.));
#14479=DIRECTION('ref_axis',(0.,0.,-1.));
#14480=DIRECTION('center_axis',(0.,1.,0.));
#14481=DIRECTION('ref_axis',(0.,0.,-1.));
#14482=DIRECTION('',(0.,1.,0.));
#14483=DIRECTION('center_axis',(0.,-1.,0.));
#14484=DIRECTION('ref_axis',(0.,0.,-1.));
#14485=DIRECTION('center_axis',(0.,-1.,0.));
#14486=DIRECTION('ref_axis',(0.,0.,-1.));
#14487=DIRECTION('center_axis',(0.,1.,0.));
#14488=DIRECTION('ref_axis',(0.,0.,-1.));
#14489=DIRECTION('',(0.,1.,0.));
#14490=DIRECTION('center_axis',(0.,-1.,0.));
#14491=DIRECTION('ref_axis',(0.,0.,-1.));
#14492=DIRECTION('center_axis',(0.,-1.,0.));
#14493=DIRECTION('ref_axis',(0.,0.,-1.));
#14494=DIRECTION('center_axis',(0.,1.,0.));
#14495=DIRECTION('ref_axis',(0.,0.,-1.));
#14496=DIRECTION('',(0.,1.,0.));
#14497=DIRECTION('center_axis',(0.,-1.,0.));
#14498=DIRECTION('ref_axis',(0.,0.,-1.));
#14499=DIRECTION('center_axis',(0.,-1.,0.));
#14500=DIRECTION('ref_axis',(0.,0.,-1.));
#14501=DIRECTION('center_axis',(0.,1.,0.));
#14502=DIRECTION('ref_axis',(0.,0.,-1.));
#14503=DIRECTION('',(0.,1.,0.));
#14504=DIRECTION('center_axis',(0.,-1.,0.));
#14505=DIRECTION('ref_axis',(0.,0.,-1.));
#14506=DIRECTION('center_axis',(0.,-1.,0.));
#14507=DIRECTION('ref_axis',(0.,0.,-1.));
#14508=DIRECTION('center_axis',(0.,1.,0.));
#14509=DIRECTION('ref_axis',(0.,0.,-1.));
#14510=DIRECTION('',(0.,1.,0.));
#14511=DIRECTION('center_axis',(0.,-1.,0.));
#14512=DIRECTION('ref_axis',(0.,0.,-1.));
#14513=DIRECTION('center_axis',(0.,-1.,0.));
#14514=DIRECTION('ref_axis',(0.,0.,-1.));
#14515=DIRECTION('center_axis',(0.,1.,0.));
#14516=DIRECTION('ref_axis',(0.,0.,-1.));
#14517=DIRECTION('',(0.,1.,0.));
#14518=DIRECTION('center_axis',(0.,-1.,0.));
#14519=DIRECTION('ref_axis',(0.,0.,-1.));
#14520=DIRECTION('center_axis',(0.,-1.,0.));
#14521=DIRECTION('ref_axis',(0.,0.,-1.));
#14522=DIRECTION('center_axis',(0.,1.,0.));
#14523=DIRECTION('ref_axis',(0.,0.,-1.));
#14524=DIRECTION('',(0.,1.,0.));
#14525=DIRECTION('center_axis',(0.,-1.,0.));
#14526=DIRECTION('ref_axis',(0.,0.,-1.));
#18751=CARTESIAN_POINT('',(0.,0.,0.));
#18752=CARTESIAN_POINT('Origin',(-6.,0.,-11.));
#18753=CARTESIAN_POINT('',(-6.,0.,-12.25));
#18754=CARTESIAN_POINT('Origin',(-6.,0.,-11.));
#18755=CARTESIAN_POINT('',(-6.,2.,-12.25));
#18756=CARTESIAN_POINT('',(-6.,0.,-12.25));
#18757=CARTESIAN_POINT('Origin',(-6.,2.,-11.));
#18758=CARTESIAN_POINT('Origin',(-11.,0.,6.));
#18759=CARTESIAN_POINT('',(-11.,0.,4.75));
#18760=CARTESIAN_POINT('Origin',(-11.,0.,6.));
#18761=CARTESIAN_POINT('',(-11.,2.,4.75));
#18762=CARTESIAN_POINT('',(-11.,0.,4.75));
#18763=CARTESIAN_POINT('Origin',(-11.,2.,6.));
#18764=CARTESIAN_POINT('Origin',(6.,0.,11.));
#18765=CARTESIAN_POINT('',(6.,0.,9.75));
#18766=CARTESIAN_POINT('Origin',(6.,0.,11.));
#18767=CARTESIAN_POINT('',(6.,2.,9.75));
#18768=CARTESIAN_POINT('',(6.,0.,9.75));
#18769=CARTESIAN_POINT('Origin',(6.,2.,11.));
#18770=CARTESIAN_POINT('Origin',(11.,0.,-6.));
#18771=CARTESIAN_POINT('',(11.,0.,-7.25));
#18772=CARTESIAN_POINT('Origin',(11.,0.,-6.));
#18773=CARTESIAN_POINT('',(11.,2.,-7.25));
#18774=CARTESIAN_POINT('',(11.,0.,-7.25));
#18775=CARTESIAN_POINT('Origin',(11.,2.,-6.));
#18776=CARTESIAN_POINT('Origin',(-11.,10.74803620541,-6.));
#18777=CARTESIAN_POINT('',(-11.,2.,-4.975));
#18778=CARTESIAN_POINT('Origin',(-11.,2.,-6.));
#18779=CARTESIAN_POINT('',(-11.,0.325,-4.975));
#18780=CARTESIAN_POINT('',(-11.,10.74803620541,-4.975));
#18781=CARTESIAN_POINT('Origin',(-11.,0.325000000000001,-6.));
#18782=CARTESIAN_POINT('Origin',(-6.,10.74803620541,11.));
#18783=CARTESIAN_POINT('',(-6.,2.,12.025));
#18784=CARTESIAN_POINT('Origin',(-6.,2.,11.));
#18785=CARTESIAN_POINT('',(-6.,0.325,12.025));
#18786=CARTESIAN_POINT('',(-6.,10.74803620541,12.025));
#18787=CARTESIAN_POINT('Origin',(-6.,0.325000000000001,11.));
#18788=CARTESIAN_POINT('Origin',(11.,10.74803620541,6.));
#18789=CARTESIAN_POINT('',(11.,2.,7.025));
#18790=CARTESIAN_POINT('Origin',(11.,2.,6.));
#18791=CARTESIAN_POINT('',(11.,0.325,7.025));
#18792=CARTESIAN_POINT('',(11.,10.74803620541,7.025));
#18793=CARTESIAN_POINT('Origin',(11.,0.325000000000001,6.));
#18794=CARTESIAN_POINT('Origin',(6.,10.74803620541,-11.));
#18795=CARTESIAN_POINT('',(6.,2.,-9.975));
#18796=CARTESIAN_POINT('Origin',(6.,2.,-11.));
#18797=CARTESIAN_POINT('',(6.,0.325,-9.975));
#18798=CARTESIAN_POINT('',(6.,10.74803620541,-9.975));
#18799=CARTESIAN_POINT('Origin',(6.,0.325000000000001,-11.));
#18800=CARTESIAN_POINT('Origin',(3.5,0.,-8.));
#18801=CARTESIAN_POINT('',(3.5,0.,-9.25));
#18802=CARTESIAN_POINT('Origin',(3.5,0.,-8.));
#18803=CARTESIAN_POINT('',(3.5,2.,-9.25));
#18804=CARTESIAN_POINT('',(3.5,0.,-9.25));
#18805=CARTESIAN_POINT('Origin',(3.5,2.,-8.));
#18806=CARTESIAN_POINT('Origin',(-8.,0.,-3.5));
#18807=CARTESIAN_POINT('',(-8.,0.,-4.75));
#18808=CARTESIAN_POINT('Origin',(-8.,0.,-3.5));
#18809=CARTESIAN_POINT('',(-8.,2.,-4.75));
#18810=CARTESIAN_POINT('',(-8.,0.,-4.75));
#18811=CARTESIAN_POINT('Origin',(-8.,2.,-3.5));
#18812=CARTESIAN_POINT('Origin',(-3.5,0.,8.));
#18813=CARTESIAN_POINT('',(-3.5,0.,6.75));
#18814=CARTESIAN_POINT('Origin',(-3.5,0.,8.));
#18815=CARTESIAN_POINT('',(-3.5,2.,6.75));
#18816=CARTESIAN_POINT('',(-3.5,0.,6.75));
#18817=CARTESIAN_POINT('Origin',(-3.5,2.,8.));
#18818=CARTESIAN_POINT('Origin',(8.,0.,3.5));
#18819=CARTESIAN_POINT('',(8.,0.,2.25));
#18820=CARTESIAN_POINT('Origin',(8.,0.,3.5));
#18821=CARTESIAN_POINT('',(8.,2.,2.25));
#18822=CARTESIAN_POINT('',(8.,0.,2.25));
#18823=CARTESIAN_POINT('Origin',(8.,2.,3.5));
#18824=CARTESIAN_POINT('Origin',(-3.5,10.74803620541,-8.));
#18825=CARTESIAN_POINT('',(-3.5,2.,-6.975));
#18826=CARTESIAN_POINT('Origin',(-3.5,2.,-8.));
#18827=CARTESIAN_POINT('',(-3.5,0.325,-6.975));
#18828=CARTESIAN_POINT('',(-3.5,10.74803620541,-6.975));
#18829=CARTESIAN_POINT('Origin',(-3.5,0.325000000000001,-8.));
#18830=CARTESIAN_POINT('Origin',(-8.,10.74803620541,3.5));
#18831=CARTESIAN_POINT('',(-8.,2.,4.525));
#18832=CARTESIAN_POINT('Origin',(-8.,2.,3.5));
#18833=CARTESIAN_POINT('',(-8.,0.325,4.525));
#18834=CARTESIAN_POINT('',(-8.,10.74803620541,4.525));
#18835=CARTESIAN_POINT('Origin',(-8.,0.325000000000001,3.5));
#18836=CARTESIAN_POINT('Origin',(3.5,10.74803620541,8.));
#18837=CARTESIAN_POINT('',(3.5,2.,9.025));
#18838=CARTESIAN_POINT('Origin',(3.5,2.,8.));
#18839=CARTESIAN_POINT('',(3.5,0.325,9.025));
#18840=CARTESIAN_POINT('',(3.5,10.74803620541,9.025));
#18841=CARTESIAN_POINT('Origin',(3.5,0.325000000000001,8.));
#18842=CARTESIAN_POINT('Origin',(8.,10.74803620541,-3.5));
#18843=CARTESIAN_POINT('',(8.,2.,-2.475));
#18844=CARTESIAN_POINT('Origin',(8.,2.,-3.5));
#18845=CARTESIAN_POINT('',(8.,0.325,-2.475));
#18846=CARTESIAN_POINT('',(8.,10.74803620541,-2.475));
#18847=CARTESIAN_POINT('Origin',(8.,0.325000000000001,-3.5));
#18848=CARTESIAN_POINT('Origin',(7.778174593052,2.,-7.778174593052));
#18849=CARTESIAN_POINT('',(7.778174593052,2.,-6.528174593052));
#18850=CARTESIAN_POINT('Origin',(7.778174593052,2.,-7.778174593052));
#18851=CARTESIAN_POINT('',(7.778174593052,0.,-6.528174593052));
#18852=CARTESIAN_POINT('',(7.778174593052,2.,-6.528174593052));
#18853=CARTESIAN_POINT('Origin',(7.778174593052,0.,-7.778174593052));
#18854=CARTESIAN_POINT('Origin',(0.,2.,-11.));
#18855=CARTESIAN_POINT('',(-1.53080849893419E-16,2.,-9.75));
#18856=CARTESIAN_POINT('Origin',(0.,2.,-11.));
#18857=CARTESIAN_POINT('',(-1.53080849893419E-16,0.,-9.75));
#18858=CARTESIAN_POINT('',(-1.53080849893419E-16,2.,-9.75));
#18859=CARTESIAN_POINT('Origin',(0.,0.,-11.));
#18860=CARTESIAN_POINT('Origin',(-7.778174593052,2.,-7.778174593052));
#18861=CARTESIAN_POINT('',(-7.778174593052,2.,-6.528174593052));
#18862=CARTESIAN_POINT('Origin',(-7.778174593052,2.,-7.778174593052));
#18863=CARTESIAN_POINT('',(-7.778174593052,0.,-6.528174593052));
#18864=CARTESIAN_POINT('',(-7.778174593052,2.,-6.528174593052));
#18865=CARTESIAN_POINT('Origin',(-7.778174593052,0.,-7.778174593052));
#18866=CARTESIAN_POINT('Origin',(-11.,2.,0.));
#18867=CARTESIAN_POINT('',(-11.,2.,1.25));
#18868=CARTESIAN_POINT('Origin',(-11.,2.,0.));
#18869=CARTESIAN_POINT('',(-11.,0.,1.25));
#18870=CARTESIAN_POINT('',(-11.,2.,1.25));
#18871=CARTESIAN_POINT('Origin',(-11.,0.,0.));
#18872=CARTESIAN_POINT('Origin',(-7.778174593052,2.,7.778174593052));
#18873=CARTESIAN_POINT('',(-7.778174593052,2.,9.028174593052));
#18874=CARTESIAN_POINT('Origin',(-7.778174593052,2.,7.778174593052));
#18875=CARTESIAN_POINT('',(-7.778174593052,0.,9.028174593052));
#18876=CARTESIAN_POINT('',(-7.778174593052,2.,9.028174593052));
#18877=CARTESIAN_POINT('Origin',(-7.778174593052,0.,7.778174593052));
#18878=CARTESIAN_POINT('Origin',(0.,2.,11.));
#18879=CARTESIAN_POINT('',(-1.53080849893419E-16,2.,12.25));
#18880=CARTESIAN_POINT('Origin',(0.,2.,11.));
#18881=CARTESIAN_POINT('',(-1.53080849893419E-16,0.,12.25));
#18882=CARTESIAN_POINT('',(-1.53080849893419E-16,2.,12.25));
#18883=CARTESIAN_POINT('Origin',(0.,0.,11.));
#18884=CARTESIAN_POINT('Origin',(7.778174593052,2.,7.778174593052));
#18885=CARTESIAN_POINT('',(7.778174593052,2.,9.028174593052));
#18886=CARTESIAN_POINT('Origin',(7.778174593052,2.,7.778174593052));
#18887=CARTESIAN_POINT('',(7.778174593052,0.,9.028174593052));
#18888=CARTESIAN_POINT('',(7.778174593052,2.,9.028174593052));
#18889=CARTESIAN_POINT('Origin',(7.778174593052,0.,7.778174593052));
#18890=CARTESIAN_POINT('Origin',(11.,2.,0.));
#18891=CARTESIAN_POINT('',(11.,2.,1.25));
#18892=CARTESIAN_POINT('Origin',(11.,2.,0.));
#18893=CARTESIAN_POINT('',(11.,0.,1.25));
#18894=CARTESIAN_POINT('',(11.,2.,1.25));
#18895=CARTESIAN_POINT('Origin',(11.,0.,0.));
#18896=CARTESIAN_POINT('Origin',(0.,1.,0.));
#18897=CARTESIAN_POINT('',(-6.12323399573677E-16,2.,5.));
#18898=CARTESIAN_POINT('Origin',(0.,2.,0.));
#18899=CARTESIAN_POINT('',(-6.12323399573677E-16,0.1999518233597,5.));
#18900=CARTESIAN_POINT('',(-6.12323399573677E-16,1.,5.));
#18901=CARTESIAN_POINT('Origin',(0.,0.1999518233597,4.25007251614318E-14));
#18902=CARTESIAN_POINT('Origin',(-11.,5.6843418860808E-11,-6.));
#18903=CARTESIAN_POINT('',(-11.,-5.68436964165642E-11,-4.64999999996962));
#18904=CARTESIAN_POINT('',(-11.,5.6843418860808E-11,-4.65000000008331));
#18905=CARTESIAN_POINT('Origin',(-11.,-5.6843418860808E-11,-6.));
#18906=CARTESIAN_POINT('Origin',(-6.,5.6843418860808E-11,11.));
#18907=CARTESIAN_POINT('',(-6.,-5.68436964165642E-11,12.3500000000304));
#18908=CARTESIAN_POINT('',(-6.,5.6843418860808E-11,12.3499999999167));
#18909=CARTESIAN_POINT('Origin',(-6.,-5.6843418860808E-11,11.));
#18910=CARTESIAN_POINT('Origin',(11.,5.6843418860808E-11,6.));
#18911=CARTESIAN_POINT('',(11.,-5.6843505617991E-11,7.35000000003038));
#18912=CARTESIAN_POINT('',(11.,5.6843418860808E-11,7.34999999991669));
#18913=CARTESIAN_POINT('Origin',(11.,-5.6843418860808E-11,6.));
#18914=CARTESIAN_POINT('Origin',(6.,5.6843418860808E-11,-11.));
#18915=CARTESIAN_POINT('',(6.,-5.68436964165642E-11,-9.64999999996962));
#18916=CARTESIAN_POINT('',(6.,5.6843418860808E-11,-9.65000000008331));
#18917=CARTESIAN_POINT('Origin',(6.,-5.6843418860808E-11,-11.));
#18918=CARTESIAN_POINT('Origin',(-3.5,5.6843418860808E-11,-8.));
#18919=CARTESIAN_POINT('',(-3.5,-5.68435576386861E-11,-6.64999999997917));
#18920=CARTESIAN_POINT('',(-3.5,5.6843418860808E-11,-6.65000000009286));
#18921=CARTESIAN_POINT('Origin',(-3.5,-5.6843418860808E-11,-8.));
#18922=CARTESIAN_POINT('Origin',(-8.,5.6843418860808E-11,3.5));
#18923=CARTESIAN_POINT('',(-8.,-5.68435569810944E-11,4.85000000002083));
#18924=CARTESIAN_POINT('',(-8.,5.6843418860808E-11,4.84999999990714));
#18925=CARTESIAN_POINT('Origin',(-8.,-5.6843418860808E-11,3.5));
#18926=CARTESIAN_POINT('Origin',(3.5,5.6843418860808E-11,8.));
#18927=CARTESIAN_POINT('',(3.5,-5.68435576386861E-11,9.35000000002083));
#18928=CARTESIAN_POINT('',(3.5,5.6843418860808E-11,9.34999999990714));
#18929=CARTESIAN_POINT('Origin',(3.5,-5.6843418860808E-11,8.));
#18930=CARTESIAN_POINT('Origin',(8.,5.6843418860808E-11,-3.5));
#18931=CARTESIAN_POINT('',(8.,-5.68435227390255E-11,-2.14999999997917));
#18932=CARTESIAN_POINT('',(8.,5.6843418860808E-11,-2.15000000009286));
#18933=CARTESIAN_POINT('Origin',(8.,-5.6843418860808E-11,-3.5));
#18934=CARTESIAN_POINT('Origin',(0.,-2.12617692341155E-5,4.25007251614318E-14));
#18935=CARTESIAN_POINT('',(-6.36810199687457E-16,-4.58884334339753E-15,
5.19994989682604));
#18936=CARTESIAN_POINT('',(-6.36812803478132E-16,-2.12617692341155E-5,5.19997115839041));
#18937=CARTESIAN_POINT('Origin',(-1.7763568394E-14,0.,0.));
#18938=CARTESIAN_POINT('Origin',(-11.,6.7,19.));
#18939=CARTESIAN_POINT('',(-9.7,6.7,19.));
#18940=CARTESIAN_POINT('Origin',(-11.,6.7,19.));
#18941=CARTESIAN_POINT('',(-9.7,6.7,17.));
#18942=CARTESIAN_POINT('',(-9.7,6.7,19.));
#18943=CARTESIAN_POINT('Origin',(-11.,6.7,17.));
#18944=CARTESIAN_POINT('Origin',(11.,6.7,19.));
#18945=CARTESIAN_POINT('',(12.3,6.7,19.));
#18946=CARTESIAN_POINT('Origin',(11.,6.7,19.));
#18947=CARTESIAN_POINT('',(12.3,6.7,17.));
#18948=CARTESIAN_POINT('',(12.3,6.7,19.));
#18949=CARTESIAN_POINT('Origin',(11.,6.7,17.));
#18950=CARTESIAN_POINT('Origin',(-18.,6.7,19.));
#18951=CARTESIAN_POINT('',(-16.7,6.7,19.));
#18952=CARTESIAN_POINT('Origin',(-18.,6.7,19.));
#18953=CARTESIAN_POINT('',(-16.7,6.7,17.));
#18954=CARTESIAN_POINT('',(-16.7,6.7,19.));
#18955=CARTESIAN_POINT('Origin',(-18.,6.7,17.));
#18956=CARTESIAN_POINT('Origin',(4.,6.7,19.));
#18957=CARTESIAN_POINT('',(5.3,6.7,19.));
#18958=CARTESIAN_POINT('Origin',(4.,6.7,19.));
#18959=CARTESIAN_POINT('',(5.3,6.7,17.));
#18960=CARTESIAN_POINT('',(5.3,6.7,19.));
#18961=CARTESIAN_POINT('Origin',(4.,6.7,17.));
#18962=CARTESIAN_POINT('Origin',(-11.,6.7,19.));
#18963=CARTESIAN_POINT('',(-9.7,6.7,-17.));
#18964=CARTESIAN_POINT('Origin',(-11.,6.7,-17.));
#18965=CARTESIAN_POINT('',(-9.7,6.7,-19.));
#18966=CARTESIAN_POINT('',(-9.7,6.7,19.));
#18967=CARTESIAN_POINT('Origin',(-11.,6.7,-19.));
#18968=CARTESIAN_POINT('Origin',(11.,6.7,19.));
#18969=CARTESIAN_POINT('',(12.3,6.7,-17.));
#18970=CARTESIAN_POINT('Origin',(11.,6.7,-17.));
#18971=CARTESIAN_POINT('',(12.3,6.7,-19.));
#18972=CARTESIAN_POINT('',(12.3,6.7,19.));
#18973=CARTESIAN_POINT('Origin',(11.,6.7,-19.));
#18974=CARTESIAN_POINT('Origin',(-18.,6.7,19.));
#18975=CARTESIAN_POINT('',(-16.7,6.7,-17.));
#18976=CARTESIAN_POINT('Origin',(-18.,6.7,-17.));
#18977=CARTESIAN_POINT('',(-16.7,6.7,-19.));
#18978=CARTESIAN_POINT('',(-16.7,6.7,19.));
#18979=CARTESIAN_POINT('Origin',(-18.,6.7,-19.));
#18980=CARTESIAN_POINT('Origin',(4.,6.7,19.));
#18981=CARTESIAN_POINT('',(5.3,6.7,-17.));
#18982=CARTESIAN_POINT('Origin',(4.,6.7,-17.));
#18983=CARTESIAN_POINT('',(5.3,6.7,-19.));
#18984=CARTESIAN_POINT('',(5.3,6.7,19.));
#18985=CARTESIAN_POINT('Origin',(4.,6.7,-19.));
#18986=CARTESIAN_POINT('Origin',(14.5,2.,16.5));
#18987=CARTESIAN_POINT('',(14.5,2.,-16.5));
#18988=CARTESIAN_POINT('',(14.5,2.,16.5));
#18989=CARTESIAN_POINT('',(14.5,2.,16.5));
#18990=CARTESIAN_POINT('',(-15.6010205144338,2.,-16.4999999999986));
#18991=CARTESIAN_POINT('',(14.5,2.,-16.5));
#18992=CARTESIAN_POINT('',(-14.5,2.,-13.03589838486));
#18993=CARTESIAN_POINT('Origin',(-20.5,2.,-13.03589838486));
#18994=CARTESIAN_POINT('',(-14.5,2.,13.03589838486));
#18995=CARTESIAN_POINT('',(-14.5,2.,16.5));
#18996=CARTESIAN_POINT('',(-15.6010205144317,2.,16.5000000000002));
#18997=CARTESIAN_POINT('Origin',(-20.5,2.,13.03589838486));
#18998=CARTESIAN_POINT('',(14.5,2.,16.5));
#18999=CARTESIAN_POINT('Origin',(14.5,2.5,16.5));
#19000=CARTESIAN_POINT('',(14.5,2.5,17.));
#19001=CARTESIAN_POINT('Origin',(14.5,2.5,16.5));
#19002=CARTESIAN_POINT('',(-17.5000000000001,2.47654106818559,16.9994493753306));
#19003=CARTESIAN_POINT('Ctrl Pts',(-17.5000096922892,2.47654352708651,16.9994494908181));
#19004=CARTESIAN_POINT('Ctrl Pts',(-17.371522845629,2.44394677638692,16.9979184348396));
#19005=CARTESIAN_POINT('Ctrl Pts',(-17.2437747299337,2.40878815792915,16.993079083846));
#19006=CARTESIAN_POINT('Ctrl Pts',(-16.9941658745484,2.33637313275275,16.9739051828542));
#19007=CARTESIAN_POINT('Ctrl Pts',(-16.8736840331451,2.29951631658164,16.9600004544787));
#19008=CARTESIAN_POINT('Ctrl Pts',(-16.6759259011892,2.2383018761184,16.9269138033769));
#19009=CARTESIAN_POINT('Ctrl Pts',(-16.5989139658977,2.21432329962625,16.9114276432015));
#19010=CARTESIAN_POINT('Ctrl Pts',(-16.4372876162009,2.1648760551481,16.8725483781765));
#19011=CARTESIAN_POINT('Ctrl Pts',(-16.3536394704351,2.13973650391793,16.8486261868388));
#19012=CARTESIAN_POINT('Ctrl Pts',(-16.1512480291796,2.08295164252046,16.7806829189119));
#19013=CARTESIAN_POINT('Ctrl Pts',(-16.0338807886608,2.05340445436661,16.7327203097712));
#19014=CARTESIAN_POINT('Ctrl Pts',(-15.8101466828132,2.01228090697128,16.6237475601439));
#19015=CARTESIAN_POINT('Ctrl Pts',(-15.7042606821881,2.00000000000037,16.5642271272144));
#19016=CARTESIAN_POINT('Ctrl Pts',(-15.60102051443,2.,16.5000000000029));
#19017=CARTESIAN_POINT('',(-17.5924003307403,2.49999999999975,17.));
#19018=CARTESIAN_POINT('Origin',(-17.5462001500739,2.63349307091694,10.8126318152261));
#19019=CARTESIAN_POINT('',(14.5,2.5,17.));
#19020=CARTESIAN_POINT('Origin',(14.5,1.,0.));
#19021=CARTESIAN_POINT('',(14.5,7.3,17.));
#19022=CARTESIAN_POINT('',(14.5,9.3,17.));
#19023=CARTESIAN_POINT('',(14.5,7.3,19.));
#19024=CARTESIAN_POINT('',(14.5,7.3,18.));
#19025=CARTESIAN_POINT('',(14.5,2.5,19.));
#19026=CARTESIAN_POINT('',(14.5,5.9,19.));
#19027=CARTESIAN_POINT('',(14.5,0.,16.5));
#19028=CARTESIAN_POINT('Origin',(14.5,2.5,16.5));
#19029=CARTESIAN_POINT('',(14.5,0.,-16.5));
#19030=CARTESIAN_POINT('',(14.5,0.,0.));
#19031=CARTESIAN_POINT('',(14.5,2.5,-19.));
#19032=CARTESIAN_POINT('Origin',(14.5,2.5,-16.5));
#19033=CARTESIAN_POINT('',(14.5,7.3,-19.));
#19034=CARTESIAN_POINT('',(14.5,5.9,-19.));
#19035=CARTESIAN_POINT('',(14.5,7.3,-17.));
#19036=CARTESIAN_POINT('',(14.5,7.3,-18.));
#19037=CARTESIAN_POINT('',(14.5,2.5,-17.));
#19038=CARTESIAN_POINT('',(14.5,2.5,-17.));
#19039=CARTESIAN_POINT('Origin',(14.5,2.5,-16.5));
#19040=CARTESIAN_POINT('Origin',(14.5,2.5,-16.5));
#19041=CARTESIAN_POINT('',(-17.59240033074,2.49999999999972,-17.));
#19042=CARTESIAN_POINT('',(14.5,2.5,-17.));
#19043=CARTESIAN_POINT('',(-17.4999999999994,2.47654106818636,-16.9994493753306));
#19044=CARTESIAN_POINT('Origin',(-17.5462001542397,2.63349226331312,-10.8126669805471));
#19045=CARTESIAN_POINT('Ctrl Pts',(-15.6010120234613,2.0000000000279,-16.4999947176331));
#19046=CARTESIAN_POINT('Ctrl Pts',(-15.704076554021,2.00000000002768,-16.5641125785337));
#19047=CARTESIAN_POINT('Ctrl Pts',(-15.8097881082795,2.01223958419737,-16.6235460520593));
#19048=CARTESIAN_POINT('Ctrl Pts',(-16.0331149291658,2.05323764858778,-16.7323757326034));
#19049=CARTESIAN_POINT('Ctrl Pts',(-16.1502586572613,2.08269792549789,-16.78029277891));
#19050=CARTESIAN_POINT('Ctrl Pts',(-16.3522616768077,2.13933342892633,-16.8482037730104));
#19051=CARTESIAN_POINT('Ctrl Pts',(-16.435747260524,2.16441192529145,-16.8721268381227));
#19052=CARTESIAN_POINT('Ctrl Pts',(-16.5973270171487,2.21383152604932,-16.9110908172613));
#19053=CARTESIAN_POINT('Ctrl Pts',(-16.6744641820304,2.23784785033491,-16.926638975002));
#19054=CARTESIAN_POINT('Ctrl Pts',(-16.8725510272894,2.29916800021421,-16.9598573262036));
#19055=CARTESIAN_POINT('Ctrl Pts',(-16.9932348770165,2.33609618849181,-16.9738155944474));
#19056=CARTESIAN_POINT('Ctrl Pts',(-17.2432994237094,2.4086572889119,-16.9930611081183));
#19057=CARTESIAN_POINT('Ctrl Pts',(-17.3712742011148,2.44388369598067,-16.997915471985));
#19058=CARTESIAN_POINT('Ctrl Pts',(-17.4999999999993,2.47654106818655,-16.9994493753306));
#19059=CARTESIAN_POINT('Origin',(-20.5,1.,-13.03589838486));
#19060=CARTESIAN_POINT('',(-15.6010205144335,1.36338022765876,-16.4999999999975));
#19061=CARTESIAN_POINT('',(-15.6010205144335,1.,-16.4999999999975));
#19062=CARTESIAN_POINT('',(-15.6010205144328,-2.57498015965307E-16,-16.4999999999996));
#19063=CARTESIAN_POINT('',(-15.6010205144335,1.,-16.4999999999975));
#19064=CARTESIAN_POINT('',(-14.5,0.,-13.03589838486));
#19065=CARTESIAN_POINT('Origin',(-20.5,0.,-13.03589838486));
#19066=CARTESIAN_POINT('',(-14.5,1.,-13.03589838486));
#19067=CARTESIAN_POINT('Origin',(-14.5,1.,0.));
#19068=CARTESIAN_POINT('',(-14.5,0.,13.03589838486));
#19069=CARTESIAN_POINT('',(-14.5,0.,0.));
#19070=CARTESIAN_POINT('',(-14.5,1.,13.03589838486));
#19071=CARTESIAN_POINT('Origin',(-20.5,1.,13.03589838486));
#19072=CARTESIAN_POINT('',(-15.6010205144326,0.,16.5));
#19073=CARTESIAN_POINT('Origin',(-20.5,0.,13.03589838486));
#19074=CARTESIAN_POINT('',(-15.6010205144335,1.36338022760973,16.4999999999975));
#19075=CARTESIAN_POINT('',(-15.6010205144335,1.,16.4999999999975));
#19076=CARTESIAN_POINT('',(-15.6010205144335,1.,16.4999999999975));
#19077=CARTESIAN_POINT('Origin',(14.5,0.,16.5));
#19078=CARTESIAN_POINT('',(14.5,0.,16.5));
#19079=CARTESIAN_POINT('',(14.5,0.,-16.5));
#19080=CARTESIAN_POINT('Origin',(14.5,9.3,17.));
#19081=CARTESIAN_POINT('',(-20.499999999999,4.17870345174027,17.));
#19082=CARTESIAN_POINT('',(-20.5,4.17870345174,17.));
#19083=CARTESIAN_POINT('',(-21.5,5.910754259309,17.));
#19084=CARTESIAN_POINT('Origin',(-19.5,5.910754259309,17.));
#19085=CARTESIAN_POINT('',(-21.5,7.3,17.));
#19086=CARTESIAN_POINT('',(-21.5,5.9,17.));
#19087=CARTESIAN_POINT('',(-19.5,9.3,17.));
#19088=CARTESIAN_POINT('Origin',(-19.5,7.3,17.));
#19089=CARTESIAN_POINT('',(12.5,9.3,17.));
#19090=CARTESIAN_POINT('',(14.5,9.3,17.));
#19091=CARTESIAN_POINT('Origin',(12.5,7.3,17.));
#19092=CARTESIAN_POINT('Ctrl Pts',(-15.57368086877,2.074394725501,16.48538787889));
#19093=CARTESIAN_POINT('Ctrl Pts',(-15.57368086877,1.358575011107,16.46081195141));
#19094=CARTESIAN_POINT('Ctrl Pts',(-15.57368086877,0.6427552967139,16.43623602393));
#19095=CARTESIAN_POINT('Ctrl Pts',(-15.57368086877,-0.07306441767953,16.41166009645));
#19096=CARTESIAN_POINT('Ctrl Pts',(-15.58274239264,2.074223770141,16.49027240659));
#19097=CARTESIAN_POINT('Ctrl Pts',(-15.58274239264,1.358116528257,16.47391169971));
#19098=CARTESIAN_POINT('Ctrl Pts',(-15.58274239264,0.6420092863734,16.45755099284));
#19099=CARTESIAN_POINT('Ctrl Pts',(-15.58274239264,-0.07409795551055,16.44119028597));
#19100=CARTESIAN_POINT('Ctrl Pts',(-15.71578181391,2.072990731385,16.56138770748));
#19101=CARTESIAN_POINT('Ctrl Pts',(-15.71578181391,1.35480965841,16.66463485657));
#19102=CARTESIAN_POINT('Ctrl Pts',(-15.71578181391,0.6366285854352,16.76788200567));
#19103=CARTESIAN_POINT('Ctrl Pts',(-15.71578181391,-0.08155248753949,16.87112915476));
#19104=CARTESIAN_POINT('Ctrl Pts',(-15.99393964446,2.105376743577,16.6924369233));
#19105=CARTESIAN_POINT('Ctrl Pts',(-15.99393964446,1.441665263409,17.01609396359));
#19106=CARTESIAN_POINT('Ctrl Pts',(-15.99393964446,0.7779537832405,17.33975100388));
#19107=CARTESIAN_POINT('Ctrl Pts',(-15.99393964446,0.114242303072,17.66340804417));
#19108=CARTESIAN_POINT('Ctrl Pts',(-16.44881838131,2.215365528923,16.83088989051));
#19109=CARTESIAN_POINT('Ctrl Pts',(-16.44881838131,1.736642688769,17.38740909059));
#19110=CARTESIAN_POINT('Ctrl Pts',(-16.44881838131,1.257919848614,17.94392829068));
#19111=CARTESIAN_POINT('Ctrl Pts',(-16.44881838131,0.7791970084599,18.50044749077));
#19112=CARTESIAN_POINT('Ctrl Pts',(-16.95084263786,2.351489777509,16.90776164253));
#19113=CARTESIAN_POINT('Ctrl Pts',(-16.95084263786,2.101712457026,17.59357039535));
#19114=CARTESIAN_POINT('Ctrl Pts',(-16.95084263786,1.851935136544,18.27937914817));
#19115=CARTESIAN_POINT('Ctrl Pts',(-16.95084263786,1.602157816061,18.96518790099));
#19116=CARTESIAN_POINT('Ctrl Pts',(-17.32661507613,2.442923903714,16.92408316831));
#19117=CARTESIAN_POINT('Ctrl Pts',(-17.32661507613,2.346928394752,17.63734287302));
#19118=CARTESIAN_POINT('Ctrl Pts',(-17.32661507613,2.250932885791,18.35060257774));
#19119=CARTESIAN_POINT('Ctrl Pts',(-17.32661507613,2.154937376829,19.06386228246));
#19120=CARTESIAN_POINT('Ctrl Pts',(-17.52801411637,2.486045160307,16.9256422694));
#19121=CARTESIAN_POINT('Ctrl Pts',(-17.52801411637,2.462574705493,17.64152420501));
#19122=CARTESIAN_POINT('Ctrl Pts',(-17.52801411637,2.439104250679,18.35740614061));
#19123=CARTESIAN_POINT('Ctrl Pts',(-17.52801411637,2.415633795865,19.07328807622));
#19124=CARTESIAN_POINT('Ctrl Pts',(-17.54206971761,2.489025840479,16.92571861498));
#19125=CARTESIAN_POINT('Ctrl Pts',(-17.54206971761,2.470568551048,17.64172895517));
#19126=CARTESIAN_POINT('Ctrl Pts',(-17.54206971761,2.452111261618,18.35773929537));
#19127=CARTESIAN_POINT('Ctrl Pts',(-17.54206971761,2.433653972188,19.07374963557));
#19128=CARTESIAN_POINT('',(-17.5000000000011,2.38270534092832,18.997246876653));
#19129=CARTESIAN_POINT('Ctrl Pts',(-17.5000000000025,2.3827053409272,18.997246876653));
#19130=CARTESIAN_POINT('Ctrl Pts',(-17.397451060852,2.25262345741567,18.9911369840666));
#19131=CARTESIAN_POINT('Ctrl Pts',(-17.2994815869931,2.11974254320617,18.9746723858667));
#19132=CARTESIAN_POINT('Ctrl Pts',(-17.1063203414114,1.84656919417232,18.9173138353435));
#19133=CARTESIAN_POINT('Ctrl Pts',(-17.0118909483542,1.70674986776022,18.8754495661767));
#19134=CARTESIAN_POINT('Ctrl Pts',(-16.7261430930788,1.27301150209775,18.7014226944282));
#19135=CARTESIAN_POINT('Ctrl Pts',(-16.5505973550705,0.992649551630207,
18.5227840186769));
#19136=CARTESIAN_POINT('Ctrl Pts',(-16.2367523912556,0.527853643828902,
18.0679946901261));
#19137=CARTESIAN_POINT('Ctrl Pts',(-16.0994701412667,0.34318463629694,17.8048543793107));
#19138=CARTESIAN_POINT('Ctrl Pts',(-15.9050156967339,0.144535698373065,
17.35458171012));
#19139=CARTESIAN_POINT('Ctrl Pts',(-15.8415060003331,0.0917554854890558,
17.192532833357));
#19140=CARTESIAN_POINT('Ctrl Pts',(-15.7177863268808,0.0189111127370208,
16.8536222157515));
#19141=CARTESIAN_POINT('Ctrl Pts',(-15.6580928898842,3.85744012468713E-14,
16.6775275456278));
#19142=CARTESIAN_POINT('Ctrl Pts',(-15.6010205144309,-5.42101086242752E-16,
16.5000000000006));
#19143=CARTESIAN_POINT('',(-17.5000000000002,2.42961219547292,17.9985825134344));
#19144=CARTESIAN_POINT('Ctrl Pts',(-17.54192267438,2.48899465693,-16.9257178151));
#19145=CARTESIAN_POINT('Ctrl Pts',(-17.54192267438,2.470484920314,-17.64172681));
#19146=CARTESIAN_POINT('Ctrl Pts',(-17.54192267438,2.451975183698,-18.3577358049));
#19147=CARTESIAN_POINT('Ctrl Pts',(-17.54192267438,2.433465447082,-19.0737447998));
#19148=CARTESIAN_POINT('Ctrl Pts',(-17.52791631184,2.486024219187,-16.92564151185));
#19149=CARTESIAN_POINT('Ctrl Pts',(-17.52791631184,2.462518543788,-17.64152217335));
#19150=CARTESIAN_POINT('Ctrl Pts',(-17.52791631184,2.43901286839,-18.35740283484));
#19151=CARTESIAN_POINT('Ctrl Pts',(-17.52791631184,2.415507192992,-19.07328349634));
#19152=CARTESIAN_POINT('Ctrl Pts',(-17.32656780917,2.44291240257,-16.92408111528));
#19153=CARTESIAN_POINT('Ctrl Pts',(-17.32656780917,2.346897549991,-17.63733736705));
#19154=CARTESIAN_POINT('Ctrl Pts',(-17.32656780917,2.250882697412,-18.35059361882));
#19155=CARTESIAN_POINT('Ctrl Pts',(-17.32656780917,2.154867844833,-19.06384987059));
#19156=CARTESIAN_POINT('Ctrl Pts',(-16.95084263786,2.351489777509,-16.90776164253));
#19157=CARTESIAN_POINT('Ctrl Pts',(-16.95084263786,2.101712457026,-17.59357039535));
#19158=CARTESIAN_POINT('Ctrl Pts',(-16.95084263786,1.851935136544,-18.27937914817));
#19159=CARTESIAN_POINT('Ctrl Pts',(-16.95084263786,1.602157816061,-18.96518790099));
#19160=CARTESIAN_POINT('Ctrl Pts',(-16.44881838131,2.215365528923,-16.83088989051));
#19161=CARTESIAN_POINT('Ctrl Pts',(-16.44881838131,1.736642688769,-17.38740909059));
#19162=CARTESIAN_POINT('Ctrl Pts',(-16.44881838131,1.257919848614,-17.94392829068));
#19163=CARTESIAN_POINT('Ctrl Pts',(-16.44881838131,0.7791970084599,-18.50044749077));
#19164=CARTESIAN_POINT('Ctrl Pts',(-15.99393964446,2.105376743577,-16.6924369233));
#19165=CARTESIAN_POINT('Ctrl Pts',(-15.99393964446,1.441665263409,-17.01609396359));
#19166=CARTESIAN_POINT('Ctrl Pts',(-15.99393964446,0.7779537832405,-17.33975100388));
#19167=CARTESIAN_POINT('Ctrl Pts',(-15.99393964446,0.114242303072,-17.66340804417));
#19168=CARTESIAN_POINT('Ctrl Pts',(-15.71573553238,2.072985342811,-16.56136590274));
#19169=CARTESIAN_POINT('Ctrl Pts',(-15.71573553238,1.354795206866,-16.66457637875));
#19170=CARTESIAN_POINT('Ctrl Pts',(-15.71573553238,0.6366050709221,-16.76778685476));
#19171=CARTESIAN_POINT('Ctrl Pts',(-15.71573553238,-0.08158506502212,-16.87099733077));
#19172=CARTESIAN_POINT('Ctrl Pts',(-15.58265688292,2.074224564534,-16.49022669701));
#19173=CARTESIAN_POINT('Ctrl Pts',(-15.58265688292,1.358118658728,-16.47378911183));
#19174=CARTESIAN_POINT('Ctrl Pts',(-15.58265688292,0.6420127529222,-16.45735152665));
#19175=CARTESIAN_POINT('Ctrl Pts',(-15.58265688292,-0.07409315288371,-16.44091394148));
#19176=CARTESIAN_POINT('Ctrl Pts',(-15.5735533349,2.07439713734,-16.48531913027));
#19177=CARTESIAN_POINT('Ctrl Pts',(-15.5735533349,1.358581479386,-16.46062757543));
#19178=CARTESIAN_POINT('Ctrl Pts',(-15.5735533349,0.6427658214313,-16.43593602058));
#19179=CARTESIAN_POINT('Ctrl Pts',(-15.5735533349,-0.07304983652298,-16.41124446574));
#19180=CARTESIAN_POINT('',(-17.4999999999994,2.38270534092991,-18.9972468766531));
#19181=CARTESIAN_POINT('',(-17.4999999999987,2.42961219547651,-17.9985825134353));
#19182=CARTESIAN_POINT('Ctrl Pts',(-15.6010205144307,1.25767452008319E-15,
-16.5000000000003));
#19183=CARTESIAN_POINT('Ctrl Pts',(-15.6579985049851,2.17455779774946E-14,
-16.6772339549203));
#19184=CARTESIAN_POINT('Ctrl Pts',(-15.7175892974837,0.0188486066689643,
-16.8530406318105));
#19185=CARTESIAN_POINT('Ctrl Pts',(-15.841088915592,0.0914580806764069,
-17.1914308410855));
#19186=CARTESIAN_POINT('Ctrl Pts',(-15.9044838682972,0.144072067619024,
-17.3532507311179));
#19187=CARTESIAN_POINT('Ctrl Pts',(-16.0985790100571,0.342122917384096,
-17.8029799327834));
#19188=CARTESIAN_POINT('Ctrl Pts',(-16.2356039725905,0.526266781326162,
-18.0659091363647));
#19189=CARTESIAN_POINT('Ctrl Pts',(-16.5490224816406,0.990195424858404,
-18.5209523776298));
#19190=CARTESIAN_POINT('Ctrl Pts',(-16.7244456612409,1.27033612063607,-18.6999333325823));
#19191=CARTESIAN_POINT('Ctrl Pts',(-17.0103210025318,1.70441228965547,-18.8747029432739));
#19192=CARTESIAN_POINT('Ctrl Pts',(-17.1050393851134,1.8447164026833,-18.9168433193197));
#19193=CARTESIAN_POINT('Ctrl Pts',(-17.2988175722228,2.11884247458825,-18.974560464731));
#19194=CARTESIAN_POINT('Ctrl Pts',(-17.3971035117738,2.25218259631596,-18.9911162770022));
#19195=CARTESIAN_POINT('Ctrl Pts',(-17.4999999999985,2.38270534093059,-18.9972468766531));
#19196=CARTESIAN_POINT('Origin',(14.5,2.5,-17.));
#19197=CARTESIAN_POINT('',(-21.5,7.3,-17.));
#19198=CARTESIAN_POINT('',(-19.5,9.3,-17.));
#19199=CARTESIAN_POINT('Origin',(-19.5,7.3,-17.));
#19200=CARTESIAN_POINT('',(-21.5,5.910754259309,-17.));
#19201=CARTESIAN_POINT('',(-21.5,5.9,-17.));
#19202=CARTESIAN_POINT('',(-20.4999999999993,4.17870345173968,-17.));
#19203=CARTESIAN_POINT('Origin',(-19.5,5.910754259309,-17.));
#19204=CARTESIAN_POINT('',(-17.59240033074,2.5,-17.));
#19205=CARTESIAN_POINT('',(12.5,9.3,-17.));
#19206=CARTESIAN_POINT('Origin',(12.5,7.3,-17.));
#19207=CARTESIAN_POINT('',(14.5,9.3,-17.));
#19208=CARTESIAN_POINT('Origin',(14.5,2.5,16.5));
#19209=CARTESIAN_POINT('',(-17.5924003307403,2.4999999999995,19.));
#19210=CARTESIAN_POINT('',(14.5,2.5,19.));
#19211=CARTESIAN_POINT('Origin',(-17.546200165371,2.53637972596203,14.9500703324677));
#19212=CARTESIAN_POINT('Origin',(14.5,2.5,-16.5));
#19213=CARTESIAN_POINT('',(-17.5924003307402,2.49999999999858,-19.));
#19214=CARTESIAN_POINT('Origin',(-17.5462001653617,2.5363797259711,-14.9500703323505));
#19215=CARTESIAN_POINT('',(14.5,2.5,-19.));
#19216=CARTESIAN_POINT('Origin',(-19.54620016537,3.628026860465,18.));
#19217=CARTESIAN_POINT('',(-20.4999999999993,4.17870345174128,19.));
#19218=CARTESIAN_POINT('',(-19.54620016537,3.628026860465,19.));
#19219=CARTESIAN_POINT('',(-20.4999999999993,4.17870345174126,18.));
#19220=CARTESIAN_POINT('',(-17.5924003307406,2.49999999999901,17.6366197724371));
#19221=CARTESIAN_POINT('',(-17.5924003307406,2.49999999999901,18.));
#19222=CARTESIAN_POINT('',(-17.5924003307406,2.49999999999901,18.));
#19223=CARTESIAN_POINT('Origin',(-19.5,5.910754259309,16.91739728962));
#19224=CARTESIAN_POINT('',(-21.5,5.910754259309,19.));
#19225=CARTESIAN_POINT('Origin',(-19.5,5.910754259309,19.));
#19226=CARTESIAN_POINT('',(-21.5,5.910754259309,16.91739728962));
#19227=CARTESIAN_POINT('Origin',(-19.5,7.3,16.91739728962));
#19228=CARTESIAN_POINT('',(-21.5,7.3,19.));
#19229=CARTESIAN_POINT('',(-21.5,7.3,16.91739728962));
#19230=CARTESIAN_POINT('',(-19.5,9.3,19.));
#19231=CARTESIAN_POINT('Origin',(-19.5,7.3,19.));
#19232=CARTESIAN_POINT('',(-19.5,9.3,16.91739728962));
#19233=CARTESIAN_POINT('Origin',(-3.5,9.3,18.));
#19234=CARTESIAN_POINT('',(12.5,9.3,19.));
#19235=CARTESIAN_POINT('',(-3.5,9.3,19.));
#19236=CARTESIAN_POINT('',(12.5,9.3,18.));
#19237=CARTESIAN_POINT('Origin',(12.5,7.3,16.91739728962));
#19238=CARTESIAN_POINT('Origin',(12.5,7.3,19.));
#19239=CARTESIAN_POINT('Ctrl Pts',(-17.42814205157,2.464509271523,16.92437907463));
#19240=CARTESIAN_POINT('Ctrl Pts',(-17.42814205157,2.404830934618,17.63798058348));
#19241=CARTESIAN_POINT('Ctrl Pts',(-17.42814205157,2.345152597712,18.35158209233));
#19242=CARTESIAN_POINT('Ctrl Pts',(-17.42814205157,2.285474260807,19.06518360117));
#19243=CARTESIAN_POINT('Ctrl Pts',(-17.45209470105,2.469672618979,16.92481104223));
#19244=CARTESIAN_POINT('Ctrl Pts',(-17.45209470105,2.418676549309,17.63913891283));
#19245=CARTESIAN_POINT('Ctrl Pts',(-17.45209470105,2.367680479639,18.35346678343));
#19246=CARTESIAN_POINT('Ctrl Pts',(-17.45209470105,2.316684409969,19.06779465403));
#19247=CARTESIAN_POINT('Ctrl Pts',(-17.50684746077,2.481493415089,16.92558269389));
#19248=CARTESIAN_POINT('Ctrl Pts',(-17.50684746077,2.450374239556,17.64120811149));
#19249=CARTESIAN_POINT('Ctrl Pts',(-17.50684746077,2.419255064023,18.35683352909));
#19250=CARTESIAN_POINT('Ctrl Pts',(-17.50684746077,2.38813588849,19.07245894669));
#19251=CARTESIAN_POINT('Ctrl Pts',(-17.58555286997,2.498518773752,16.92598231066));
#19252=CARTESIAN_POINT('Ctrl Pts',(-17.58555286997,2.496028063562,17.64227969147));
#19253=CARTESIAN_POINT('Ctrl Pts',(-17.58555286997,2.493537353372,18.35857707229));
#19254=CARTESIAN_POINT('Ctrl Pts',(-17.58555286997,2.491046643181,19.0748744531));
#19255=CARTESIAN_POINT('Ctrl Pts',(-17.6403056297,2.510362756466,16.92576611527));
#19256=CARTESIAN_POINT('Ctrl Pts',(-17.6403056297,2.527787929129,17.64169995942));
#19257=CARTESIAN_POINT('Ctrl Pts',(-17.6403056297,2.545213101792,18.35763380357));
#19258=CARTESIAN_POINT('Ctrl Pts',(-17.6403056297,2.562638274455,19.07356764772));
#19259=CARTESIAN_POINT('Ctrl Pts',(-17.66425827917,2.515540684786,16.92557687661));
#19260=CARTESIAN_POINT('Ctrl Pts',(-17.66425827917,2.541672642685,17.64119251234));
#19261=CARTESIAN_POINT('Ctrl Pts',(-17.66425827917,2.567804600584,18.35680814807));
#19262=CARTESIAN_POINT('Ctrl Pts',(-17.66425827917,2.593936558484,19.0724237838));
#19263=CARTESIAN_POINT('Ctrl Pts',(-17.42814205157,2.464509271523,-16.92437907463));
#19264=CARTESIAN_POINT('Ctrl Pts',(-17.42814205157,2.404830934618,-17.63798058348));
#19265=CARTESIAN_POINT('Ctrl Pts',(-17.42814205157,2.345152597712,-18.35158209233));
#19266=CARTESIAN_POINT('Ctrl Pts',(-17.42814205157,2.285474260807,-19.06518360117));
#19267=CARTESIAN_POINT('Ctrl Pts',(-17.45209470105,2.469672618979,-16.92481104223));
#19268=CARTESIAN_POINT('Ctrl Pts',(-17.45209470105,2.418676549309,-17.63913891283));
#19269=CARTESIAN_POINT('Ctrl Pts',(-17.45209470105,2.367680479639,-18.35346678343));
#19270=CARTESIAN_POINT('Ctrl Pts',(-17.45209470105,2.316684409969,-19.06779465403));
#19271=CARTESIAN_POINT('Ctrl Pts',(-17.50684746077,2.481493415089,-16.92558269389));
#19272=CARTESIAN_POINT('Ctrl Pts',(-17.50684746077,2.450374239556,-17.64120811149));
#19273=CARTESIAN_POINT('Ctrl Pts',(-17.50684746077,2.419255064023,-18.35683352909));
#19274=CARTESIAN_POINT('Ctrl Pts',(-17.50684746077,2.38813588849,-19.07245894669));
#19275=CARTESIAN_POINT('Ctrl Pts',(-17.58555286997,2.498518773752,-16.92598231066));
#19276=CARTESIAN_POINT('Ctrl Pts',(-17.58555286997,2.496028063562,-17.64227969147));
#19277=CARTESIAN_POINT('Ctrl Pts',(-17.58555286997,2.493537353372,-18.35857707229));
#19278=CARTESIAN_POINT('Ctrl Pts',(-17.58555286997,2.491046643181,-19.0748744531));
#19279=CARTESIAN_POINT('Ctrl Pts',(-17.6403056297,2.510362756466,-16.92576611527));
#19280=CARTESIAN_POINT('Ctrl Pts',(-17.6403056297,2.527787929129,-17.64169995942));
#19281=CARTESIAN_POINT('Ctrl Pts',(-17.6403056297,2.545213101792,-18.35763380357));
#19282=CARTESIAN_POINT('Ctrl Pts',(-17.6403056297,2.562638274455,-19.07356764772));
#19283=CARTESIAN_POINT('Ctrl Pts',(-17.66425827917,2.515540684786,-16.92557687661));
#19284=CARTESIAN_POINT('Ctrl Pts',(-17.66425827917,2.541672642685,-17.64119251234));
#19285=CARTESIAN_POINT('Ctrl Pts',(-17.66425827917,2.567804600584,-18.35680814807));
#19286=CARTESIAN_POINT('Ctrl Pts',(-17.66425827917,2.593936558484,-19.0724237838));
#19287=CARTESIAN_POINT('',(-17.5924003307402,2.49999999999784,-17.636619772437));
#19288=CARTESIAN_POINT('',(-17.5924003307402,2.49999999999716,-18.0000000145074));
#19289=CARTESIAN_POINT('',(-17.5924003307402,2.49999999999716,-18.0000000145074));
#19290=CARTESIAN_POINT('Origin',(-3.5,9.3,-18.));
#19291=CARTESIAN_POINT('',(-19.5,9.3,-19.));
#19292=CARTESIAN_POINT('',(-19.5,9.3,-18.));
#19293=CARTESIAN_POINT('',(12.5,9.3,-19.));
#19294=CARTESIAN_POINT('',(12.5,9.3,-18.));
#19295=CARTESIAN_POINT('',(-3.5,9.3,-19.));
#19296=CARTESIAN_POINT('Origin',(-19.5,7.3,-16.91739728962));
#19297=CARTESIAN_POINT('',(-21.5,7.3,-19.));
#19298=CARTESIAN_POINT('Origin',(-19.5,7.3,-19.));
#19299=CARTESIAN_POINT('',(-21.5,7.3,-16.91739728962));
#19300=CARTESIAN_POINT('Origin',(-19.5,5.910754259309,-16.91739728962));
#19301=CARTESIAN_POINT('',(-21.5,5.910754259309,-19.));
#19302=CARTESIAN_POINT('',(-21.5,5.910754259309,-16.91739728962));
#19303=CARTESIAN_POINT('',(-20.4999999999997,4.1787034517407,-19.));
#19304=CARTESIAN_POINT('Origin',(-19.5,5.910754259309,-19.));
#19305=CARTESIAN_POINT('',(-20.5,4.17870345174009,-16.91739728962));
#19306=CARTESIAN_POINT('Origin',(-19.54620016537,3.628026860465,-18.));
#19307=CARTESIAN_POINT('',(-19.54620016537,3.628026860465,-19.));
#19308=CARTESIAN_POINT('Origin',(12.5,7.3,-16.91739728962));
#19309=CARTESIAN_POINT('Origin',(12.5,7.3,-19.));
#19310=CARTESIAN_POINT('Origin',(14.5,9.3,19.));
#19311=CARTESIAN_POINT('',(-21.5,9.3,19.));
#19312=CARTESIAN_POINT('Origin',(14.5,2.5,-19.));
#19313=CARTESIAN_POINT('',(-21.5,2.5,-19.));
#19314=CARTESIAN_POINT('Origin',(-21.5,5.9,18.));
#19315=CARTESIAN_POINT('Origin',(-21.5,5.9,-18.));
#19316=CARTESIAN_POINT('Origin',(8.,10.74803620541,-3.5));
#19317=CARTESIAN_POINT('',(8.,0.1,-2.25));
#19318=CARTESIAN_POINT('Origin',(8.,0.0999999999999994,-3.5));
#19319=CARTESIAN_POINT('',(8.,2.,-2.25));
#19320=CARTESIAN_POINT('',(8.,10.74803620541,-2.25));
#19321=CARTESIAN_POINT('Origin',(8.,2.,-3.5));
#19322=CARTESIAN_POINT('Origin',(3.5,10.74803620541,8.));
#19323=CARTESIAN_POINT('',(3.5,0.1,9.25));
#19324=CARTESIAN_POINT('Origin',(3.5,0.0999999999999994,8.));
#19325=CARTESIAN_POINT('',(3.5,2.,9.25));
#19326=CARTESIAN_POINT('',(3.5,10.74803620541,9.25));
#19327=CARTESIAN_POINT('Origin',(3.5,2.,8.));
#19328=CARTESIAN_POINT('Origin',(-8.,10.74803620541,3.5));
#19329=CARTESIAN_POINT('',(-8.,0.1,4.75));
#19330=CARTESIAN_POINT('Origin',(-8.,0.0999999999999994,3.5));
#19331=CARTESIAN_POINT('',(-8.,2.,4.75));
#19332=CARTESIAN_POINT('',(-8.,10.74803620541,4.75));
#19333=CARTESIAN_POINT('Origin',(-8.,2.,3.5));
#19334=CARTESIAN_POINT('Origin',(-3.5,10.74803620541,-8.));
#19335=CARTESIAN_POINT('',(-3.5,0.1,-6.75));
#19336=CARTESIAN_POINT('Origin',(-3.5,0.0999999999999994,-8.));
#19337=CARTESIAN_POINT('',(-3.5,2.,-6.75));
#19338=CARTESIAN_POINT('',(-3.5,10.74803620541,-6.75));
#19339=CARTESIAN_POINT('Origin',(-3.5,2.,-8.));
#19340=CARTESIAN_POINT('Origin',(6.,10.74803620541,-11.));
#19341=CARTESIAN_POINT('',(6.,0.1,-9.75));
#19342=CARTESIAN_POINT('Origin',(6.,0.0999999999999994,-11.));
#19343=CARTESIAN_POINT('',(6.,2.,-9.75));
#19344=CARTESIAN_POINT('',(6.,10.74803620541,-9.75));
#19345=CARTESIAN_POINT('Origin',(6.,2.,-11.));
#19346=CARTESIAN_POINT('Origin',(11.,10.74803620541,6.));
#19347=CARTESIAN_POINT('',(11.,0.1,7.25));
#19348=CARTESIAN_POINT('Origin',(11.,0.0999999999999994,6.));
#19349=CARTESIAN_POINT('',(11.,2.,7.25));
#19350=CARTESIAN_POINT('',(11.,10.74803620541,7.25));
#19351=CARTESIAN_POINT('Origin',(11.,2.,6.));
#19352=CARTESIAN_POINT('Origin',(-6.,10.74803620541,11.));
#19353=CARTESIAN_POINT('',(-6.,0.1,12.25));
#19354=CARTESIAN_POINT('Origin',(-6.,0.0999999999999994,11.));
#19355=CARTESIAN_POINT('',(-6.,2.,12.25));
#19356=CARTESIAN_POINT('',(-6.,10.74803620541,12.25));
#19357=CARTESIAN_POINT('Origin',(-6.,2.,11.));
#19358=CARTESIAN_POINT('Origin',(-11.,10.74803620541,-6.));
#19359=CARTESIAN_POINT('',(-11.,0.1,-4.75));
#19360=CARTESIAN_POINT('Origin',(-11.,0.0999999999999994,-6.));
#19361=CARTESIAN_POINT('',(-11.,2.,-4.75));
#19362=CARTESIAN_POINT('',(-11.,10.74803620541,-4.75));
#19363=CARTESIAN_POINT('Origin',(-11.,2.,-6.));
#20148=UNCERTAINTY_MEASURE_WITH_UNIT(LENGTH_MEASURE(0.01),#20177,
'DISTANCE_ACCURACY_VALUE',
'Maximum model space distance between geometric entities at asserted c
onnectivities');
#20160=UNCERTAINTY_MEASURE_WITH_UNIT(LENGTH_MEASURE(0.01),#20177,
'DISTANCE_ACCURACY_VALUE',
'Maximum model space distance between geometric entities at asserted c
onnectivities');
#20164=(
GEOMETRIC_REPRESENTATION_CONTEXT(3)
GLOBAL_UNCERTAINTY_ASSIGNED_CONTEXT((#20148))
GLOBAL_UNIT_ASSIGNED_CONTEXT((#20177,#20179,#20180))
REPRESENTATION_CONTEXT('','3D')
);
#20176=(
GEOMETRIC_REPRESENTATION_CONTEXT(3)
GLOBAL_UNCERTAINTY_ASSIGNED_CONTEXT((#20160))
GLOBAL_UNIT_ASSIGNED_CONTEXT((#20177,#20179,#20180))
REPRESENTATION_CONTEXT('','3D')
);
#20177=(
LENGTH_UNIT()
NAMED_UNIT(*)
SI_UNIT(.MILLI.,.METRE.)
);
#20179=(
NAMED_UNIT(*)
PLANE_ANGLE_UNIT()
SI_UNIT($,.RADIAN.)
);
#20180=(
NAMED_UNIT(*)
SI_UNIT($,.STERADIAN.)
SOLID_ANGLE_UNIT()
);
#20184=SHAPE_DEFINITION_REPRESENTATION(#20199,#20258);
#20199=PRODUCT_DEFINITION_SHAPE('',$,#20274);
#20258=SHAPE_REPRESENTATION('',(#11674,#195,#196,#197,#198,#199,#200,#201,
#202),#20164);
#20270=PRODUCT_DEFINITION_CONTEXT('part definition',#20317,'design');
#20274=PRODUCT_DEFINITION('Servo Frame','Servo Frame',#20289,#20270);
#20289=PRODUCT_DEFINITION_FORMATION('',$,#20322);
#20317=APPLICATION_CONTEXT(
'Core Data for Automotive Mechanical Design Process');
#20318=PRODUCT_CONTEXT('part definition',#20317,'mechanical');
#20322=PRODUCT('Servo Frame','Servo Frame',$,(#20318));
#20334=PRESENTATION_STYLE_ASSIGNMENT((#20339));
#20339=SURFACE_STYLE_USAGE(.BOTH.,#20344);
#20344=SURFACE_SIDE_STYLE('',(#20349));
#20349=SURFACE_STYLE_FILL_AREA(#20354);
#20354=FILL_AREA_STYLE('Steel - Satin',(#20359));
#20359=FILL_AREA_STYLE_COLOUR('Steel - Satin',#20364);
#20364=COLOUR_RGB('Steel - Satin',0.627450980392157,0.627450980392157,0.627450980392157);
ENDSEC;
END-ISO-10303-21;
